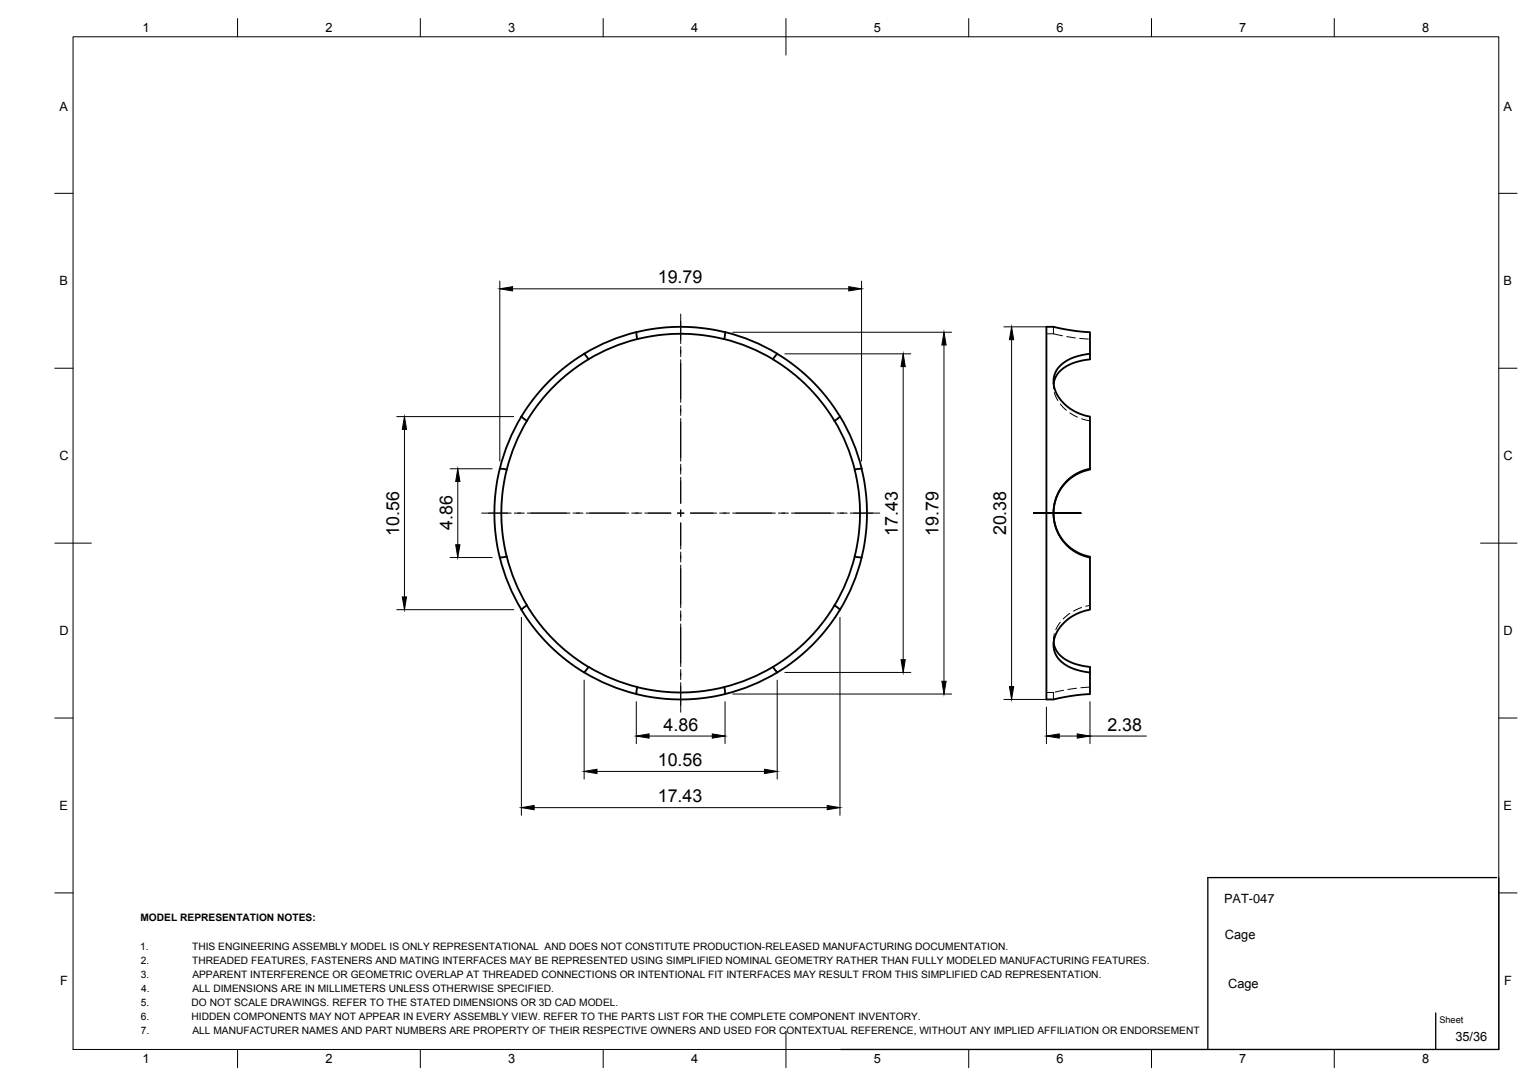
ISO-10303-21;
HEADER;
/* Generated by software containing ST-Developer
 * from STEP Tools, Inc. (www.steptools.com) 
 */

FILE_DESCRIPTION(
/* description */ ('Gravity roller conveyor section'),
/* implementation_level */ '2;1');

FILE_NAME(
/* name */ 'Cage.step',
/* time_stamp */ '2026-11-02T07:43:02-08:00',
/* author */ (''),
/* organization */ (''),
/* preprocessor_version */ 'ST-DEVELOPER v20.2',
/* originating_system */ 'Autodesk Translation Framework v15.17.0.0',
/* authorisation */ '');

FILE_SCHEMA (('AUTOMOTIVE_DESIGN { 1 0 10303 214 3 1 1 }'));
ENDSEC;

DATA;
#10=MECHANICAL_DESIGN_GEOMETRIC_PRESENTATION_REPRESENTATION('',(#562),#13821);
#397=SPHERICAL_SURFACE('',#8542,0.247676);
#398=SPHERICAL_SURFACE('',#8558,0.247676);
#399=SPHERICAL_SURFACE('',#8563,0.247676);
#400=SPHERICAL_SURFACE('',#8568,0.247676);
#401=SPHERICAL_SURFACE('',#8573,0.247676);
#402=SPHERICAL_SURFACE('',#8578,0.247676);
#403=SPHERICAL_SURFACE('',#8583,0.247676);
#404=SPHERICAL_SURFACE('',#8591,0.247676);
#443=B_SPLINE_CURVE_WITH_KNOTS('',3,(#12876,#12877,#12878,#12879,#12880,
#12881,#12882,#12883,#12884,#12885,#12886,#12887,#12888,#12889,#12890,#12891,
#12892,#12893,#12894,#12895,#12896,#12897),.UNSPECIFIED.,.F.,.F.,(4,2,2,
2,2,2,2,2,2,2,4),(0.0473477652366656,0.126350602536658,0.189525903804987,
0.252701205073317,0.313298422430275,0.373895639787233,0.434492857144191,
0.495090074501149,0.558265375769478,0.621440677037807,0.7004435143378),
 .UNSPECIFIED.);
#444=B_SPLINE_CURVE_WITH_KNOTS('',3,(#12901,#12902,#12903,#12904,#12905,
#12906,#12907,#12908,#12909,#12910,#12911,#12912,#12913,#12914,#12915,#12916,
#12917,#12918,#12919,#12920,#12921,#12922),.UNSPECIFIED.,.F.,.F.,(4,2,2,
2,2,2,2,2,2,2,4),(0.0464897534940957,0.0852567806515119,0.170513561303024,
0.246687263103517,0.308657850341199,0.370628437578881,0.432599024816563,
0.494569612054245,0.570743313854739,0.656000094506251,0.694767121663666),
 .UNSPECIFIED.);
#445=B_SPLINE_CURVE_WITH_KNOTS('',3,(#12928,#12929,#12930,#12931,#12932,
#12933,#12934,#12935,#12936,#12937,#12938,#12939,#12940,#12941,#12942,#12943,
#12944,#12945,#12946,#12947,#12948,#12949),.UNSPECIFIED.,.F.,.F.,(4,2,2,
2,2,2,2,2,2,2,4),(0.0464897534940957,0.0852567806515118,0.170513561303024,
0.246687263103517,0.308657850341199,0.370628437578881,0.432599024816563,
0.494569612054245,0.570743313854738,0.65600009450625,0.694767121663666),
 .UNSPECIFIED.);
#446=B_SPLINE_CURVE_WITH_KNOTS('',3,(#12953,#12954,#12955,#12956,#12957,
#12958,#12959,#12960,#12961,#12962,#12963,#12964,#12965,#12966,#12967,#12968,
#12969,#12970,#12971,#12972,#12973,#12974),.UNSPECIFIED.,.F.,.F.,(4,2,2,
2,2,2,2,2,2,2,4),(0.0464897534940957,0.0852567806515119,0.170513561303024,
0.246687263103517,0.308657850341199,0.370628437578881,0.432599024816563,
0.494569612054245,0.570743313854739,0.656000094506251,0.694767121663666),
 .UNSPECIFIED.);
#447=B_SPLINE_CURVE_WITH_KNOTS('',3,(#12978,#12979,#12980,#12981,#12982,
#12983,#12984,#12985,#12986,#12987,#12988,#12989),.UNSPECIFIED.,.F.,.F.,
(4,2,2,2,2,4),(0.0464897534940957,0.0852567806515119,0.170513561303024,
0.246687263103517,0.308657850341199,0.370628437578881),.UNSPECIFIED.);
#448=B_SPLINE_CURVE_WITH_KNOTS('',3,(#12994,#12995,#12996,#12997,#12998,
#12999,#13000,#13001,#13002,#13003,#13004,#13005),.UNSPECIFIED.,.F.,.F.,
(4,2,2,2,2,4),(0.370628437578881,0.432599024816563,0.494569612054245,0.570743313854738,
0.65600009450625,0.694767121663666),.UNSPECIFIED.);
#449=B_SPLINE_CURVE_WITH_KNOTS('',3,(#13009,#13010,#13011,#13012,#13013,
#13014,#13015,#13016,#13017,#13018,#13019,#13020,#13021,#13022,#13023,#13024,
#13025,#13026,#13027,#13028,#13029,#13030),.UNSPECIFIED.,.F.,.F.,(4,2,2,
2,2,2,2,2,2,2,4),(0.0464897534940957,0.0852567806515121,0.170513561303024,
0.246687263103518,0.308657850341199,0.370628437578881,0.432599024816563,
0.494569612054245,0.570743313854738,0.65600009450625,0.694767121663666),
 .UNSPECIFIED.);
#450=B_SPLINE_CURVE_WITH_KNOTS('',3,(#13034,#13035,#13036,#13037,#13038,
#13039,#13040,#13041,#13042,#13043,#13044,#13045,#13046,#13047,#13048,#13049,
#13050,#13051,#13052,#13053,#13054,#13055),.UNSPECIFIED.,.F.,.F.,(4,2,2,
2,2,2,2,2,2,2,4),(0.0464897534940957,0.0852567806515119,0.170513561303024,
0.246687263103517,0.308657850341199,0.370628437578881,0.432599024816563,
0.494569612054245,0.570743313854738,0.65600009450625,0.694767121663667),
 .UNSPECIFIED.);
#451=B_SPLINE_CURVE_WITH_KNOTS('',3,(#13059,#13060,#13061,#13062,#13063,
#13064,#13065,#13066,#13067,#13068,#13069,#13070,#13071,#13072,#13073,#13074,
#13075,#13076,#13077,#13078,#13079,#13080),.UNSPECIFIED.,.F.,.F.,(4,2,2,
2,2,2,2,2,2,2,4),(0.0464897534940957,0.0852567806515119,0.170513561303024,
0.246687263103517,0.308657850341199,0.370628437578881,0.432599024816563,
0.494569612054245,0.570743313854738,0.65600009450625,0.694767121663666),
 .UNSPECIFIED.);
#452=B_SPLINE_CURVE_WITH_KNOTS('',3,(#13084,#13085,#13086,#13087,#13088,
#13089,#13090,#13091,#13092,#13093,#13094,#13095,#13096,#13097,#13098,#13099,
#13100,#13101,#13102,#13103,#13104,#13105),.UNSPECIFIED.,.F.,.F.,(4,2,2,
2,2,2,2,2,2,2,4),(0.0464897534940957,0.0852567806515119,0.170513561303024,
0.246687263103517,0.308657850341199,0.370628437578881,0.432599024816563,
0.494569612054245,0.570743313854739,0.656000094506251,0.694767121663667),
 .UNSPECIFIED.);
#453=B_SPLINE_CURVE_WITH_KNOTS('',3,(#13113,#13114,#13115,#13116,#13117,
#13118,#13119,#13120,#13121,#13122,#13123,#13124,#13125,#13126,#13127,#13128,
#13129,#13130,#13131,#13132,#13133,#13134),.UNSPECIFIED.,.F.,.F.,(4,2,2,
2,2,2,2,2,2,2,4),(0.0473477652366656,0.126350602536658,0.189525903804987,
0.252701205073316,0.313298422430274,0.373895639787232,0.434492857144191,
0.495090074501149,0.558265375769478,0.621440677037807,0.7004435143378),
 .UNSPECIFIED.);
#454=B_SPLINE_CURVE_WITH_KNOTS('',3,(#13142,#13143,#13144,#13145,#13146,
#13147,#13148,#13149,#13150,#13151,#13152,#13153,#13154,#13155,#13156,#13157,
#13158,#13159,#13160,#13161,#13162,#13163),.UNSPECIFIED.,.F.,.F.,(4,2,2,
2,2,2,2,2,2,2,4),(0.0473477652366656,0.126350602536658,0.189525903804987,
0.252701205073317,0.313298422430275,0.373895639787233,0.434492857144191,
0.495090074501149,0.558265375769478,0.621440677037807,0.7004435143378),
 .UNSPECIFIED.);
#455=B_SPLINE_CURVE_WITH_KNOTS('',3,(#13172,#13173,#13174,#13175,#13176,
#13177,#13178,#13179,#13180,#13181,#13182,#13183),.UNSPECIFIED.,.F.,.F.,
(4,2,2,2,2,4),(0.0473477652366656,0.126350602536658,0.189525903804987,0.252701205073316,
0.313298422430275,0.373895639787233),.UNSPECIFIED.);
#456=B_SPLINE_CURVE_WITH_KNOTS('',3,(#13185,#13186,#13187,#13188,#13189,
#13190,#13191,#13192,#13193,#13194,#13195,#13196),.UNSPECIFIED.,.F.,.F.,
(4,2,2,2,2,4),(0.373895639787233,0.434492857144191,0.495090074501149,0.558265375769478,
0.621440677037807,0.7004435143378),.UNSPECIFIED.);
#457=B_SPLINE_CURVE_WITH_KNOTS('',3,(#13203,#13204,#13205,#13206,#13207,
#13208,#13209,#13210,#13211,#13212,#13213,#13214,#13215,#13216,#13217,#13218,
#13219,#13220,#13221,#13222,#13223,#13224),.UNSPECIFIED.,.F.,.F.,(4,2,2,
2,2,2,2,2,2,2,4),(0.0473477652366656,0.126350602536658,0.189525903804987,
0.252701205073316,0.313298422430275,0.373895639787233,0.434492857144191,
0.495090074501149,0.558265375769478,0.621440677037807,0.7004435143378),
 .UNSPECIFIED.);
#458=B_SPLINE_CURVE_WITH_KNOTS('',3,(#13232,#13233,#13234,#13235,#13236,
#13237,#13238,#13239,#13240,#13241,#13242,#13243,#13244,#13245,#13246,#13247,
#13248,#13249,#13250,#13251,#13252,#13253),.UNSPECIFIED.,.F.,.F.,(4,2,2,
2,2,2,2,2,2,2,4),(0.0473477652366656,0.126350602536658,0.189525903804987,
0.252701205073317,0.313298422430275,0.373895639787233,0.434492857144191,
0.495090074501149,0.558265375769478,0.621440677037807,0.7004435143378),
 .UNSPECIFIED.);
#459=B_SPLINE_CURVE_WITH_KNOTS('',3,(#13261,#13262,#13263,#13264,#13265,
#13266,#13267,#13268,#13269,#13270,#13271,#13272,#13273,#13274,#13275,#13276,
#13277,#13278,#13279,#13280,#13281,#13282),.UNSPECIFIED.,.F.,.F.,(4,2,2,
2,2,2,2,2,2,2,4),(0.0473477652366656,0.126350602536658,0.189525903804987,
0.252701205073316,0.313298422430275,0.373895639787233,0.434492857144191,
0.495090074501149,0.558265375769478,0.621440677037807,0.7004435143378),
 .UNSPECIFIED.);
#460=B_SPLINE_CURVE_WITH_KNOTS('',3,(#13291,#13292,#13293,#13294,#13295,
#13296,#13297,#13298,#13299,#13300,#13301,#13302,#13303,#13304,#13305,#13306,
#13307,#13308,#13309,#13310,#13311,#13312),.UNSPECIFIED.,.F.,.F.,(4,2,2,
2,2,2,2,2,2,2,4),(0.0473477652366656,0.126350602536658,0.189525903804987,
0.252701205073317,0.313298422430275,0.373895639787233,0.434492857144191,
0.495090074501149,0.558265375769478,0.621440677037807,0.7004435143378),
 .UNSPECIFIED.);
#487=SHAPE_REPRESENTATION_RELATIONSHIP('SRR','None',#14026,#521);
#521=ADVANCED_BREP_SHAPE_REPRESENTATION('',(#602),#13813);
#562=STYLED_ITEM('',(#14190),#602);
#602=MANIFOLD_SOLID_BREP('Continuous crown cage',#7662);
#682=FACE_BOUND('',#1842,.T.);
#947=PLANE('',#8555);
#948=PLANE('',#8560);
#949=PLANE('',#8565);
#950=PLANE('',#8570);
#951=PLANE('',#8575);
#952=PLANE('',#8580);
#953=PLANE('',#8589);
#954=PLANE('',#8593);
#955=PLANE('',#8594);
#1332=FACE_OUTER_BOUND('',#1824,.T.);
#1333=FACE_OUTER_BOUND('',#1825,.T.);
#1334=FACE_OUTER_BOUND('',#1826,.T.);
#1335=FACE_OUTER_BOUND('',#1827,.T.);
#1336=FACE_OUTER_BOUND('',#1828,.T.);
#1337=FACE_OUTER_BOUND('',#1829,.T.);
#1338=FACE_OUTER_BOUND('',#1830,.T.);
#1339=FACE_OUTER_BOUND('',#1831,.T.);
#1340=FACE_OUTER_BOUND('',#1832,.T.);
#1341=FACE_OUTER_BOUND('',#1833,.T.);
#1342=FACE_OUTER_BOUND('',#1834,.T.);
#1343=FACE_OUTER_BOUND('',#1835,.T.);
#1344=FACE_OUTER_BOUND('',#1836,.T.);
#1345=FACE_OUTER_BOUND('',#1837,.T.);
#1346=FACE_OUTER_BOUND('',#1838,.T.);
#1347=FACE_OUTER_BOUND('',#1839,.T.);
#1348=FACE_OUTER_BOUND('',#1840,.T.);
#1349=FACE_OUTER_BOUND('',#1841,.T.);
#1350=FACE_OUTER_BOUND('',#1843,.T.);
#1824=EDGE_LOOP('',(#6722,#6723,#6724,#6725));
#1825=EDGE_LOOP('',(#6726,#6727,#6728,#6729,#6730,#6731,#6732,#6733,#6734,
#6735,#6736,#6737,#6738,#6739,#6740,#6741,#6742,#6743,#6744,#6745));
#1826=EDGE_LOOP('',(#6746,#6747,#6748,#6749));
#1827=EDGE_LOOP('',(#6750,#6751,#6752,#6753));
#1828=EDGE_LOOP('',(#6754,#6755,#6756,#6757));
#1829=EDGE_LOOP('',(#6758,#6759,#6760,#6761));
#1830=EDGE_LOOP('',(#6762,#6763,#6764,#6765));
#1831=EDGE_LOOP('',(#6766,#6767,#6768,#6769,#6770,#6771));
#1832=EDGE_LOOP('',(#6772,#6773,#6774,#6775));
#1833=EDGE_LOOP('',(#6776,#6777,#6778,#6779));
#1834=EDGE_LOOP('',(#6780,#6781,#6782,#6783));
#1835=EDGE_LOOP('',(#6784,#6785,#6786,#6787));
#1836=EDGE_LOOP('',(#6788,#6789,#6790,#6791));
#1837=EDGE_LOOP('',(#6792,#6793,#6794,#6795));
#1838=EDGE_LOOP('',(#6796,#6797,#6798,#6799,#6800,#6801,#6802,#6803,#6804,
#6805,#6806,#6807,#6808,#6809,#6810,#6811,#6812,#6813,#6814,#6815));
#1839=EDGE_LOOP('',(#6816,#6817,#6818,#6819));
#1840=EDGE_LOOP('',(#6820,#6821,#6822,#6823));
#1841=EDGE_LOOP('',(#6824));
#1842=EDGE_LOOP('',(#6825));
#1843=EDGE_LOOP('',(#6826,#6827,#6828,#6829));
#2550=LINE('',#12991,#3268);
#2551=LINE('',#13287,#3269);
#3268=VECTOR('',#10431,1.019052);
#3269=VECTOR('',#10508,0.980948);
#3512=CIRCLE('',#8543,0.243053047864041);
#3513=CIRCLE('',#8544,0.243053047864041);
#3514=CIRCLE('',#8546,1.019052);
#3515=CIRCLE('',#8547,1.019052);
#3516=CIRCLE('',#8548,1.019052);
#3517=CIRCLE('',#8549,1.019052);
#3518=CIRCLE('',#8550,1.019052);
#3519=CIRCLE('',#8551,1.019052);
#3520=CIRCLE('',#8552,1.019052);
#3521=CIRCLE('',#8553,1.019052);
#3522=CIRCLE('',#8554,1.019052);
#3523=CIRCLE('',#8556,0.980948);
#3524=CIRCLE('',#8557,0.243053047864041);
#3525=CIRCLE('',#8559,0.243053047864041);
#3526=CIRCLE('',#8561,0.980948);
#3527=CIRCLE('',#8562,0.243053047864041);
#3528=CIRCLE('',#8564,0.243053047864041);
#3529=CIRCLE('',#8566,0.980948);
#3530=CIRCLE('',#8567,0.243053047864041);
#3531=CIRCLE('',#8569,0.243053047864041);
#3532=CIRCLE('',#8571,0.980948);
#3533=CIRCLE('',#8572,0.243053047864041);
#3534=CIRCLE('',#8574,0.243053047864041);
#3535=CIRCLE('',#8576,0.980948);
#3536=CIRCLE('',#8577,0.243053047864041);
#3537=CIRCLE('',#8579,0.243053047864041);
#3538=CIRCLE('',#8581,0.980948);
#3539=CIRCLE('',#8582,0.243053047864041);
#3540=CIRCLE('',#8584,0.243053047864041);
#3541=CIRCLE('',#8586,0.980948);
#3542=CIRCLE('',#8587,0.980948);
#3543=CIRCLE('',#8588,0.980948);
#3544=CIRCLE('',#8590,0.243053047864041);
#3545=CIRCLE('',#8592,0.243053047864041);
#4104=VERTEX_POINT('',#12874);
#4105=VERTEX_POINT('',#12875);
#4106=VERTEX_POINT('',#12898);
#4107=VERTEX_POINT('',#12900);
#4108=VERTEX_POINT('',#12925);
#4109=VERTEX_POINT('',#12927);
#4110=VERTEX_POINT('',#12950);
#4111=VERTEX_POINT('',#12952);
#4112=VERTEX_POINT('',#12975);
#4113=VERTEX_POINT('',#12977);
#4114=VERTEX_POINT('',#12990);
#4115=VERTEX_POINT('',#12993);
#4116=VERTEX_POINT('',#13006);
#4117=VERTEX_POINT('',#13008);
#4118=VERTEX_POINT('',#13031);
#4119=VERTEX_POINT('',#13033);
#4120=VERTEX_POINT('',#13056);
#4121=VERTEX_POINT('',#13058);
#4122=VERTEX_POINT('',#13081);
#4123=VERTEX_POINT('',#13083);
#4124=VERTEX_POINT('',#13108);
#4125=VERTEX_POINT('',#13112);
#4126=VERTEX_POINT('',#13137);
#4127=VERTEX_POINT('',#13141);
#4128=VERTEX_POINT('',#13166);
#4129=VERTEX_POINT('',#13170);
#4130=VERTEX_POINT('',#13171);
#4131=VERTEX_POINT('',#13198);
#4132=VERTEX_POINT('',#13202);
#4133=VERTEX_POINT('',#13227);
#4134=VERTEX_POINT('',#13231);
#4135=VERTEX_POINT('',#13256);
#4136=VERTEX_POINT('',#13260);
#4137=VERTEX_POINT('',#13285);
#4138=VERTEX_POINT('',#13288);
#4139=VERTEX_POINT('',#13290);
#4998=EDGE_CURVE('',#4104,#4105,#443,.T.);
#4999=EDGE_CURVE('',#4106,#4104,#3512,.T.);
#5000=EDGE_CURVE('',#4107,#4106,#444,.T.);
#5001=EDGE_CURVE('',#4105,#4107,#3513,.T.);
#5002=EDGE_CURVE('',#4108,#4106,#3514,.T.);
#5003=EDGE_CURVE('',#4108,#4109,#445,.T.);
#5004=EDGE_CURVE('',#4110,#4109,#3515,.T.);
#5005=EDGE_CURVE('',#4110,#4111,#446,.T.);
#5006=EDGE_CURVE('',#4112,#4111,#3516,.T.);
#5007=EDGE_CURVE('',#4112,#4113,#447,.T.);
#5008=EDGE_CURVE('',#4113,#4114,#2550,.T.);
#5009=EDGE_CURVE('',#4114,#4114,#3517,.T.);
#5010=EDGE_CURVE('',#4113,#4115,#448,.T.);
#5011=EDGE_CURVE('',#4116,#4115,#3518,.T.);
#5012=EDGE_CURVE('',#4116,#4117,#449,.T.);
#5013=EDGE_CURVE('',#4118,#4117,#3519,.T.);
#5014=EDGE_CURVE('',#4118,#4119,#450,.T.);
#5015=EDGE_CURVE('',#4120,#4119,#3520,.T.);
#5016=EDGE_CURVE('',#4120,#4121,#451,.T.);
#5017=EDGE_CURVE('',#4122,#4121,#3521,.T.);
#5018=EDGE_CURVE('',#4122,#4123,#452,.T.);
#5019=EDGE_CURVE('',#4107,#4123,#3522,.T.);
#5020=EDGE_CURVE('',#4104,#4124,#3523,.T.);
#5021=EDGE_CURVE('',#4124,#4108,#3524,.T.);
#5022=EDGE_CURVE('',#4125,#4124,#453,.T.);
#5023=EDGE_CURVE('',#4109,#4125,#3525,.T.);
#5024=EDGE_CURVE('',#4125,#4126,#3526,.T.);
#5025=EDGE_CURVE('',#4126,#4110,#3527,.T.);
#5026=EDGE_CURVE('',#4127,#4126,#454,.T.);
#5027=EDGE_CURVE('',#4111,#4127,#3528,.T.);
#5028=EDGE_CURVE('',#4127,#4128,#3529,.T.);
#5029=EDGE_CURVE('',#4128,#4112,#3530,.T.);
#5030=EDGE_CURVE('',#4129,#4130,#455,.T.);
#5031=EDGE_CURVE('',#4115,#4129,#3531,.T.);
#5032=EDGE_CURVE('',#4130,#4128,#456,.T.);
#5033=EDGE_CURVE('',#4129,#4131,#3532,.T.);
#5034=EDGE_CURVE('',#4131,#4116,#3533,.T.);
#5035=EDGE_CURVE('',#4132,#4131,#457,.T.);
#5036=EDGE_CURVE('',#4117,#4132,#3534,.T.);
#5037=EDGE_CURVE('',#4132,#4133,#3535,.T.);
#5038=EDGE_CURVE('',#4133,#4118,#3536,.T.);
#5039=EDGE_CURVE('',#4134,#4133,#458,.T.);
#5040=EDGE_CURVE('',#4119,#4134,#3537,.T.);
#5041=EDGE_CURVE('',#4134,#4135,#3538,.T.);
#5042=EDGE_CURVE('',#4135,#4120,#3539,.T.);
#5043=EDGE_CURVE('',#4136,#4135,#459,.T.);
#5044=EDGE_CURVE('',#4121,#4136,#3540,.T.);
#5045=EDGE_CURVE('',#4137,#4137,#3541,.T.);
#5046=EDGE_CURVE('',#4137,#4130,#2551,.T.);
#5047=EDGE_CURVE('',#4138,#4105,#3542,.T.);
#5048=EDGE_CURVE('',#4138,#4139,#460,.T.);
#5049=EDGE_CURVE('',#4136,#4139,#3543,.T.);
#5050=EDGE_CURVE('',#4123,#4138,#3544,.T.);
#5051=EDGE_CURVE('',#4139,#4122,#3545,.T.);
#6722=ORIENTED_EDGE('',*,*,#4998,.F.);
#6723=ORIENTED_EDGE('',*,*,#4999,.F.);
#6724=ORIENTED_EDGE('',*,*,#5000,.F.);
#6725=ORIENTED_EDGE('',*,*,#5001,.F.);
#6726=ORIENTED_EDGE('',*,*,#5000,.T.);
#6727=ORIENTED_EDGE('',*,*,#5002,.F.);
#6728=ORIENTED_EDGE('',*,*,#5003,.T.);
#6729=ORIENTED_EDGE('',*,*,#5004,.F.);
#6730=ORIENTED_EDGE('',*,*,#5005,.T.);
#6731=ORIENTED_EDGE('',*,*,#5006,.F.);
#6732=ORIENTED_EDGE('',*,*,#5007,.T.);
#6733=ORIENTED_EDGE('',*,*,#5008,.T.);
#6734=ORIENTED_EDGE('',*,*,#5009,.F.);
#6735=ORIENTED_EDGE('',*,*,#5008,.F.);
#6736=ORIENTED_EDGE('',*,*,#5010,.T.);
#6737=ORIENTED_EDGE('',*,*,#5011,.F.);
#6738=ORIENTED_EDGE('',*,*,#5012,.T.);
#6739=ORIENTED_EDGE('',*,*,#5013,.F.);
#6740=ORIENTED_EDGE('',*,*,#5014,.T.);
#6741=ORIENTED_EDGE('',*,*,#5015,.F.);
#6742=ORIENTED_EDGE('',*,*,#5016,.T.);
#6743=ORIENTED_EDGE('',*,*,#5017,.F.);
#6744=ORIENTED_EDGE('',*,*,#5018,.T.);
#6745=ORIENTED_EDGE('',*,*,#5019,.F.);
#6746=ORIENTED_EDGE('',*,*,#4999,.T.);
#6747=ORIENTED_EDGE('',*,*,#5020,.T.);
#6748=ORIENTED_EDGE('',*,*,#5021,.T.);
#6749=ORIENTED_EDGE('',*,*,#5002,.T.);
#6750=ORIENTED_EDGE('',*,*,#5022,.F.);
#6751=ORIENTED_EDGE('',*,*,#5023,.F.);
#6752=ORIENTED_EDGE('',*,*,#5003,.F.);
#6753=ORIENTED_EDGE('',*,*,#5021,.F.);
#6754=ORIENTED_EDGE('',*,*,#5023,.T.);
#6755=ORIENTED_EDGE('',*,*,#5024,.T.);
#6756=ORIENTED_EDGE('',*,*,#5025,.T.);
#6757=ORIENTED_EDGE('',*,*,#5004,.T.);
#6758=ORIENTED_EDGE('',*,*,#5026,.F.);
#6759=ORIENTED_EDGE('',*,*,#5027,.F.);
#6760=ORIENTED_EDGE('',*,*,#5005,.F.);
#6761=ORIENTED_EDGE('',*,*,#5025,.F.);
#6762=ORIENTED_EDGE('',*,*,#5027,.T.);
#6763=ORIENTED_EDGE('',*,*,#5028,.T.);
#6764=ORIENTED_EDGE('',*,*,#5029,.T.);
#6765=ORIENTED_EDGE('',*,*,#5006,.T.);
#6766=ORIENTED_EDGE('',*,*,#5030,.F.);
#6767=ORIENTED_EDGE('',*,*,#5031,.F.);
#6768=ORIENTED_EDGE('',*,*,#5010,.F.);
#6769=ORIENTED_EDGE('',*,*,#5007,.F.);
#6770=ORIENTED_EDGE('',*,*,#5029,.F.);
#6771=ORIENTED_EDGE('',*,*,#5032,.F.);
#6772=ORIENTED_EDGE('',*,*,#5031,.T.);
#6773=ORIENTED_EDGE('',*,*,#5033,.T.);
#6774=ORIENTED_EDGE('',*,*,#5034,.T.);
#6775=ORIENTED_EDGE('',*,*,#5011,.T.);
#6776=ORIENTED_EDGE('',*,*,#5035,.F.);
#6777=ORIENTED_EDGE('',*,*,#5036,.F.);
#6778=ORIENTED_EDGE('',*,*,#5012,.F.);
#6779=ORIENTED_EDGE('',*,*,#5034,.F.);
#6780=ORIENTED_EDGE('',*,*,#5036,.T.);
#6781=ORIENTED_EDGE('',*,*,#5037,.T.);
#6782=ORIENTED_EDGE('',*,*,#5038,.T.);
#6783=ORIENTED_EDGE('',*,*,#5013,.T.);
#6784=ORIENTED_EDGE('',*,*,#5039,.F.);
#6785=ORIENTED_EDGE('',*,*,#5040,.F.);
#6786=ORIENTED_EDGE('',*,*,#5014,.F.);
#6787=ORIENTED_EDGE('',*,*,#5038,.F.);
#6788=ORIENTED_EDGE('',*,*,#5040,.T.);
#6789=ORIENTED_EDGE('',*,*,#5041,.T.);
#6790=ORIENTED_EDGE('',*,*,#5042,.T.);
#6791=ORIENTED_EDGE('',*,*,#5015,.T.);
#6792=ORIENTED_EDGE('',*,*,#5016,.F.);
#6793=ORIENTED_EDGE('',*,*,#5042,.F.);
#6794=ORIENTED_EDGE('',*,*,#5043,.F.);
#6795=ORIENTED_EDGE('',*,*,#5044,.F.);
#6796=ORIENTED_EDGE('',*,*,#5045,.F.);
#6797=ORIENTED_EDGE('',*,*,#5046,.T.);
#6798=ORIENTED_EDGE('',*,*,#5032,.T.);
#6799=ORIENTED_EDGE('',*,*,#5028,.F.);
#6800=ORIENTED_EDGE('',*,*,#5026,.T.);
#6801=ORIENTED_EDGE('',*,*,#5024,.F.);
#6802=ORIENTED_EDGE('',*,*,#5022,.T.);
#6803=ORIENTED_EDGE('',*,*,#5020,.F.);
#6804=ORIENTED_EDGE('',*,*,#4998,.T.);
#6805=ORIENTED_EDGE('',*,*,#5047,.F.);
#6806=ORIENTED_EDGE('',*,*,#5048,.T.);
#6807=ORIENTED_EDGE('',*,*,#5049,.F.);
#6808=ORIENTED_EDGE('',*,*,#5043,.T.);
#6809=ORIENTED_EDGE('',*,*,#5041,.F.);
#6810=ORIENTED_EDGE('',*,*,#5039,.T.);
#6811=ORIENTED_EDGE('',*,*,#5037,.F.);
#6812=ORIENTED_EDGE('',*,*,#5035,.T.);
#6813=ORIENTED_EDGE('',*,*,#5033,.F.);
#6814=ORIENTED_EDGE('',*,*,#5030,.T.);
#6815=ORIENTED_EDGE('',*,*,#5046,.F.);
#6816=ORIENTED_EDGE('',*,*,#5001,.T.);
#6817=ORIENTED_EDGE('',*,*,#5019,.T.);
#6818=ORIENTED_EDGE('',*,*,#5050,.T.);
#6819=ORIENTED_EDGE('',*,*,#5047,.T.);
#6820=ORIENTED_EDGE('',*,*,#5018,.F.);
#6821=ORIENTED_EDGE('',*,*,#5051,.F.);
#6822=ORIENTED_EDGE('',*,*,#5048,.F.);
#6823=ORIENTED_EDGE('',*,*,#5050,.F.);
#6824=ORIENTED_EDGE('',*,*,#5009,.T.);
#6825=ORIENTED_EDGE('',*,*,#5045,.T.);
#6826=ORIENTED_EDGE('',*,*,#5044,.T.);
#6827=ORIENTED_EDGE('',*,*,#5049,.T.);
#6828=ORIENTED_EDGE('',*,*,#5051,.T.);
#6829=ORIENTED_EDGE('',*,*,#5017,.T.);
#7188=CYLINDRICAL_SURFACE('',#8545,1.019052);
#7189=CYLINDRICAL_SURFACE('',#8585,0.980948);
#7533=ADVANCED_FACE('',(#1332),#397,.F.);
#7534=ADVANCED_FACE('',(#1333),#7188,.T.);
#7535=ADVANCED_FACE('',(#1334),#947,.T.);
#7536=ADVANCED_FACE('',(#1335),#398,.F.);
#7537=ADVANCED_FACE('',(#1336),#948,.T.);
#7538=ADVANCED_FACE('',(#1337),#399,.F.);
#7539=ADVANCED_FACE('',(#1338),#949,.T.);
#7540=ADVANCED_FACE('',(#1339),#400,.F.);
#7541=ADVANCED_FACE('',(#1340),#950,.T.);
#7542=ADVANCED_FACE('',(#1341),#401,.F.);
#7543=ADVANCED_FACE('',(#1342),#951,.T.);
#7544=ADVANCED_FACE('',(#1343),#402,.F.);
#7545=ADVANCED_FACE('',(#1344),#952,.T.);
#7546=ADVANCED_FACE('',(#1345),#403,.F.);
#7547=ADVANCED_FACE('',(#1346),#7189,.F.);
#7548=ADVANCED_FACE('',(#1347),#953,.T.);
#7549=ADVANCED_FACE('',(#1348),#404,.F.);
#7550=ADVANCED_FACE('',(#1349,#682),#954,.T.);
#7551=ADVANCED_FACE('',(#1350),#955,.T.);
#7662=CLOSED_SHELL('',(#7533,#7534,#7535,#7536,#7537,#7538,#7539,#7540,
#7541,#7542,#7543,#7544,#7545,#7546,#7547,#7548,#7549,#7550,#7551));
#8541=AXIS2_PLACEMENT_3D('',#12872,#10415,#10416);
#8542=AXIS2_PLACEMENT_3D('',#12873,#10417,#10418);
#8543=AXIS2_PLACEMENT_3D('',#12899,#10419,#10420);
#8544=AXIS2_PLACEMENT_3D('',#12923,#10421,#10422);
#8545=AXIS2_PLACEMENT_3D('',#12924,#10423,#10424);
#8546=AXIS2_PLACEMENT_3D('',#12926,#10425,#10426);
#8547=AXIS2_PLACEMENT_3D('',#12951,#10427,#10428);
#8548=AXIS2_PLACEMENT_3D('',#12976,#10429,#10430);
#8549=AXIS2_PLACEMENT_3D('',#12992,#10432,#10433);
#8550=AXIS2_PLACEMENT_3D('',#13007,#10434,#10435);
#8551=AXIS2_PLACEMENT_3D('',#13032,#10436,#10437);
#8552=AXIS2_PLACEMENT_3D('',#13057,#10438,#10439);
#8553=AXIS2_PLACEMENT_3D('',#13082,#10440,#10441);
#8554=AXIS2_PLACEMENT_3D('',#13106,#10442,#10443);
#8555=AXIS2_PLACEMENT_3D('',#13107,#10444,#10445);
#8556=AXIS2_PLACEMENT_3D('',#13109,#10446,#10447);
#8557=AXIS2_PLACEMENT_3D('',#13110,#10448,#10449);
#8558=AXIS2_PLACEMENT_3D('',#13111,#10450,#10451);
#8559=AXIS2_PLACEMENT_3D('',#13135,#10452,#10453);
#8560=AXIS2_PLACEMENT_3D('',#13136,#10454,#10455);
#8561=AXIS2_PLACEMENT_3D('',#13138,#10456,#10457);
#8562=AXIS2_PLACEMENT_3D('',#13139,#10458,#10459);
#8563=AXIS2_PLACEMENT_3D('',#13140,#10460,#10461);
#8564=AXIS2_PLACEMENT_3D('',#13164,#10462,#10463);
#8565=AXIS2_PLACEMENT_3D('',#13165,#10464,#10465);
#8566=AXIS2_PLACEMENT_3D('',#13167,#10466,#10467);
#8567=AXIS2_PLACEMENT_3D('',#13168,#10468,#10469);
#8568=AXIS2_PLACEMENT_3D('',#13169,#10470,#10471);
#8569=AXIS2_PLACEMENT_3D('',#13184,#10472,#10473);
#8570=AXIS2_PLACEMENT_3D('',#13197,#10474,#10475);
#8571=AXIS2_PLACEMENT_3D('',#13199,#10476,#10477);
#8572=AXIS2_PLACEMENT_3D('',#13200,#10478,#10479);
#8573=AXIS2_PLACEMENT_3D('',#13201,#10480,#10481);
#8574=AXIS2_PLACEMENT_3D('',#13225,#10482,#10483);
#8575=AXIS2_PLACEMENT_3D('',#13226,#10484,#10485);
#8576=AXIS2_PLACEMENT_3D('',#13228,#10486,#10487);
#8577=AXIS2_PLACEMENT_3D('',#13229,#10488,#10489);
#8578=AXIS2_PLACEMENT_3D('',#13230,#10490,#10491);
#8579=AXIS2_PLACEMENT_3D('',#13254,#10492,#10493);
#8580=AXIS2_PLACEMENT_3D('',#13255,#10494,#10495);
#8581=AXIS2_PLACEMENT_3D('',#13257,#10496,#10497);
#8582=AXIS2_PLACEMENT_3D('',#13258,#10498,#10499);
#8583=AXIS2_PLACEMENT_3D('',#13259,#10500,#10501);
#8584=AXIS2_PLACEMENT_3D('',#13283,#10502,#10503);
#8585=AXIS2_PLACEMENT_3D('',#13284,#10504,#10505);
#8586=AXIS2_PLACEMENT_3D('',#13286,#10506,#10507);
#8587=AXIS2_PLACEMENT_3D('',#13289,#10509,#10510);
#8588=AXIS2_PLACEMENT_3D('',#13313,#10511,#10512);
#8589=AXIS2_PLACEMENT_3D('',#13314,#10513,#10514);
#8590=AXIS2_PLACEMENT_3D('',#13315,#10515,#10516);
#8591=AXIS2_PLACEMENT_3D('',#13316,#10517,#10518);
#8592=AXIS2_PLACEMENT_3D('',#13317,#10519,#10520);
#8593=AXIS2_PLACEMENT_3D('',#13318,#10521,#10522);
#8594=AXIS2_PLACEMENT_3D('',#13319,#10523,#10524);
#10415=DIRECTION('axis',(0.,0.,1.));
#10416=DIRECTION('refdir',(1.,0.,0.));
#10417=DIRECTION('center_axis',(0.,0.,1.));
#10418=DIRECTION('ref_axis',(1.,0.,0.));
#10419=DIRECTION('center_axis',(0.,-1.,0.));
#10420=DIRECTION('ref_axis',(0.,0.,-1.));
#10421=DIRECTION('center_axis',(0.,-1.,0.));
#10422=DIRECTION('ref_axis',(0.,0.,-1.));
#10423=DIRECTION('center_axis',(0.,1.,0.));
#10424=DIRECTION('ref_axis',(1.,0.,0.));
#10425=DIRECTION('center_axis',(0.,1.,0.));
#10426=DIRECTION('ref_axis',(1.,0.,0.));
#10427=DIRECTION('center_axis',(0.,1.,0.));
#10428=DIRECTION('ref_axis',(1.,0.,0.));
#10429=DIRECTION('center_axis',(0.,1.,0.));
#10430=DIRECTION('ref_axis',(1.,0.,0.));
#10431=DIRECTION('',(0.,-1.,0.));
#10432=DIRECTION('center_axis',(0.,-1.,0.));
#10433=DIRECTION('ref_axis',(1.,0.,0.));
#10434=DIRECTION('center_axis',(0.,1.,0.));
#10435=DIRECTION('ref_axis',(1.,0.,0.));
#10436=DIRECTION('center_axis',(0.,1.,0.));
#10437=DIRECTION('ref_axis',(1.,0.,0.));
#10438=DIRECTION('center_axis',(0.,1.,0.));
#10439=DIRECTION('ref_axis',(1.,0.,0.));
#10440=DIRECTION('center_axis',(0.,1.,0.));
#10441=DIRECTION('ref_axis',(1.,0.,0.));
#10442=DIRECTION('center_axis',(0.,1.,0.));
#10443=DIRECTION('ref_axis',(1.,0.,0.));
#10444=DIRECTION('center_axis',(0.,1.,0.));
#10445=DIRECTION('ref_axis',(1.,0.,0.));
#10446=DIRECTION('center_axis',(0.,-1.,0.));
#10447=DIRECTION('ref_axis',(1.,0.,0.));
#10448=DIRECTION('center_axis',(0.,-1.,0.));
#10449=DIRECTION('ref_axis',(0.,0.,-1.));
#10450=DIRECTION('center_axis',(6.12323399573677E-17,0.,1.));
#10451=DIRECTION('ref_axis',(1.,0.,0.));
#10452=DIRECTION('center_axis',(0.,-1.,0.));
#10453=DIRECTION('ref_axis',(0.,0.,-1.));
#10454=DIRECTION('center_axis',(0.,1.,0.));
#10455=DIRECTION('ref_axis',(1.,0.,0.));
#10456=DIRECTION('center_axis',(0.,-1.,0.));
#10457=DIRECTION('ref_axis',(1.,0.,0.));
#10458=DIRECTION('center_axis',(0.,-1.,0.));
#10459=DIRECTION('ref_axis',(0.,0.,-1.));
#10460=DIRECTION('center_axis',(0.,0.,1.));
#10461=DIRECTION('ref_axis',(1.,0.,0.));
#10462=DIRECTION('center_axis',(0.,-1.,0.));
#10463=DIRECTION('ref_axis',(0.,0.,-1.));
#10464=DIRECTION('center_axis',(0.,1.,0.));
#10465=DIRECTION('ref_axis',(1.,0.,0.));
#10466=DIRECTION('center_axis',(0.,-1.,0.));
#10467=DIRECTION('ref_axis',(1.,0.,0.));
#10468=DIRECTION('center_axis',(0.,-1.,0.));
#10469=DIRECTION('ref_axis',(0.,0.,-1.));
#10470=DIRECTION('center_axis',(0.,0.,1.));
#10471=DIRECTION('ref_axis',(1.,0.,0.));
#10472=DIRECTION('center_axis',(0.,-1.,0.));
#10473=DIRECTION('ref_axis',(0.,0.,-1.));
#10474=DIRECTION('center_axis',(0.,1.,0.));
#10475=DIRECTION('ref_axis',(1.,0.,0.));
#10476=DIRECTION('center_axis',(0.,-1.,0.));
#10477=DIRECTION('ref_axis',(1.,0.,0.));
#10478=DIRECTION('center_axis',(0.,-1.,0.));
#10479=DIRECTION('ref_axis',(0.,0.,-1.));
#10480=DIRECTION('center_axis',(0.,0.,1.));
#10481=DIRECTION('ref_axis',(1.,0.,0.));
#10482=DIRECTION('center_axis',(0.,-1.,0.));
#10483=DIRECTION('ref_axis',(0.,0.,-1.));
#10484=DIRECTION('center_axis',(0.,1.,0.));
#10485=DIRECTION('ref_axis',(1.,0.,0.));
#10486=DIRECTION('center_axis',(0.,-1.,0.));
#10487=DIRECTION('ref_axis',(1.,0.,0.));
#10488=DIRECTION('center_axis',(0.,-1.,0.));
#10489=DIRECTION('ref_axis',(0.,0.,-1.));
#10490=DIRECTION('center_axis',(6.12323399573676E-17,0.,1.));
#10491=DIRECTION('ref_axis',(1.,0.,0.));
#10492=DIRECTION('center_axis',(0.,-1.,0.));
#10493=DIRECTION('ref_axis',(0.,0.,-1.));
#10494=DIRECTION('center_axis',(0.,1.,0.));
#10495=DIRECTION('ref_axis',(1.,0.,0.));
#10496=DIRECTION('center_axis',(0.,-1.,0.));
#10497=DIRECTION('ref_axis',(1.,0.,0.));
#10498=DIRECTION('center_axis',(0.,-1.,0.));
#10499=DIRECTION('ref_axis',(0.,0.,-1.));
#10500=DIRECTION('center_axis',(0.,0.,1.));
#10501=DIRECTION('ref_axis',(1.,0.,0.));
#10502=DIRECTION('center_axis',(0.,-1.,0.));
#10503=DIRECTION('ref_axis',(0.,0.,-1.));
#10504=DIRECTION('center_axis',(0.,1.,0.));
#10505=DIRECTION('ref_axis',(1.,0.,0.));
#10506=DIRECTION('center_axis',(0.,1.,0.));
#10507=DIRECTION('ref_axis',(1.,0.,0.));
#10508=DIRECTION('',(0.,1.,0.));
#10509=DIRECTION('center_axis',(0.,-1.,0.));
#10510=DIRECTION('ref_axis',(1.,0.,0.));
#10511=DIRECTION('center_axis',(0.,-1.,0.));
#10512=DIRECTION('ref_axis',(1.,0.,0.));
#10513=DIRECTION('center_axis',(0.,1.,0.));
#10514=DIRECTION('ref_axis',(1.,0.,0.));
#10515=DIRECTION('center_axis',(0.,-1.,0.));
#10516=DIRECTION('ref_axis',(0.,0.,-1.));
#10517=DIRECTION('center_axis',(0.,0.,1.));
#10518=DIRECTION('ref_axis',(1.,0.,0.));
#10519=DIRECTION('center_axis',(0.,-1.,0.));
#10520=DIRECTION('ref_axis',(0.,0.,-1.));
#10521=DIRECTION('center_axis',(0.,-1.,0.));
#10522=DIRECTION('ref_axis',(-1.,0.,0.));
#10523=DIRECTION('center_axis',(0.,1.,0.));
#10524=DIRECTION('ref_axis',(1.,0.,0.));
#12872=CARTESIAN_POINT('',(0.,0.,0.));
#12873=CARTESIAN_POINT('Origin',(0.707106781186547,0.,0.707106781186548));
#12874=CARTESIAN_POINT('',(0.504455939115715,-0.04763,0.841298510752802));
#12875=CARTESIAN_POINT('',(0.841298510752802,-0.04763,0.504455939115715));
#12876=CARTESIAN_POINT('Ctrl Pts',(0.504455939115715,-0.04763,0.841298510752802));
#12877=CARTESIAN_POINT('Ctrl Pts',(0.508899795931835,-0.0740444353928835,
0.838633903678357));
#12878=CARTESIAN_POINT('Ctrl Pts',(0.517157748491652,-0.0999305678883309,
0.833661031856294));
#12879=CARTESIAN_POINT('Ctrl Pts',(0.537715343527944,-0.142345102874864,
0.820511285096538));
#12880=CARTESIAN_POINT('Ctrl Pts',(0.548874290046456,-0.159766064500479,
0.813159949759));
#12881=CARTESIAN_POINT('Ctrl Pts',(0.573915184558107,-0.190326085855194,
0.795684265985089));
#12882=CARTESIAN_POINT('Ctrl Pts',(0.587792702767295,-0.203463743702801,
0.78555112003688));
#12883=CARTESIAN_POINT('Ctrl Pts',(0.615966552324775,-0.224161999508995,
0.763642258217233));
#12884=CARTESIAN_POINT('Ctrl Pts',(0.631684198665438,-0.232861760990032,
0.750785745543687));
#12885=CARTESIAN_POINT('Ctrl Pts',(0.663382628119203,-0.244251601209411,
0.722929908501543));
#12886=CARTESIAN_POINT('Ctrl Pts',(0.679352081686668,-0.246942143572133,
0.707917883896095));
#12887=CARTESIAN_POINT('Ctrl Pts',(0.707917883896095,-0.246942143572133,
0.679352081686668));
#12888=CARTESIAN_POINT('Ctrl Pts',(0.722929908501543,-0.244251601209411,
0.663382628119203));
#12889=CARTESIAN_POINT('Ctrl Pts',(0.750785745543687,-0.232861760990032,
0.631684198665439));
#12890=CARTESIAN_POINT('Ctrl Pts',(0.763642258217232,-0.224161999508995,
0.615966552324775));
#12891=CARTESIAN_POINT('Ctrl Pts',(0.78555112003688,-0.203463743702801,
0.587792702767295));
#12892=CARTESIAN_POINT('Ctrl Pts',(0.795684265985088,-0.190326085855194,
0.573915184558108));
#12893=CARTESIAN_POINT('Ctrl Pts',(0.813159949759,-0.15976606450048,0.548874290046456));
#12894=CARTESIAN_POINT('Ctrl Pts',(0.820511285096538,-0.142345102874864,
0.537715343527944));
#12895=CARTESIAN_POINT('Ctrl Pts',(0.833661031856294,-0.099930567888331,
0.517157748491653));
#12896=CARTESIAN_POINT('Ctrl Pts',(0.838633903678357,-0.0740444353928835,
0.508899795931835));
#12897=CARTESIAN_POINT('Ctrl Pts',(0.841298510752801,-0.0476299999999999,
0.504455939115715));
#12898=CARTESIAN_POINT('',(0.528110872004958,-0.04763,0.871530771444223));
#12899=CARTESIAN_POINT('Origin',(0.707106781186547,-0.04763,0.707106781186548));
#12900=CARTESIAN_POINT('',(0.871530771444223,-0.04763,0.528110872004959));
#12901=CARTESIAN_POINT('Ctrl Pts',(0.871530771444223,-0.0476300000000001,
0.528110872004958));
#12902=CARTESIAN_POINT('Ctrl Pts',(0.87014664509073,-0.0609922781173483,
0.530395067942936));
#12903=CARTESIAN_POINT('Ctrl Pts',(0.868149331745851,-0.0742967091364493,
0.533674141594226));
#12904=CARTESIAN_POINT('Ctrl Pts',(0.85981294420286,-0.115492077056649,
0.54708917182331));
#12905=CARTESIAN_POINT('Ctrl Pts',(0.850993704737257,-0.141695629206859,
0.560922177770136));
#12906=CARTESIAN_POINT('Ctrl Pts',(0.830754510485543,-0.181890537957859,
0.590422647829571));
#12907=CARTESIAN_POINT('Ctrl Pts',(0.816896541396381,-0.201072148666545,
0.609616703125488));
#12908=CARTESIAN_POINT('Ctrl Pts',(0.792310597819928,-0.223955109275652,
0.641117951819998));
#12909=CARTESIAN_POINT('Ctrl Pts',(0.779109323683612,-0.232742381310829,
0.657208095763053));
#12910=CARTESIAN_POINT('Ctrl Pts',(0.750552691816206,-0.244234834628584,
0.68964083160521));
#12911=CARTESIAN_POINT('Ctrl Pts',(0.735185187071673,-0.246942143572133,
0.705971972091755));
#12912=CARTESIAN_POINT('Ctrl Pts',(0.705971972091754,-0.246942143572133,
0.735185187071673));
#12913=CARTESIAN_POINT('Ctrl Pts',(0.689640831605209,-0.244234834628584,
0.750552691816206));
#12914=CARTESIAN_POINT('Ctrl Pts',(0.657208095763052,-0.232742381310829,
0.779109323683612));
#12915=CARTESIAN_POINT('Ctrl Pts',(0.641117951819998,-0.223955109275652,
0.792310597819928));
#12916=CARTESIAN_POINT('Ctrl Pts',(0.609616703125487,-0.201072148666545,
0.816896541396382));
#12917=CARTESIAN_POINT('Ctrl Pts',(0.590422647829571,-0.181890537957858,
0.830754510485544));
#12918=CARTESIAN_POINT('Ctrl Pts',(0.560922177770135,-0.141695629206858,
0.850993704737257));
#12919=CARTESIAN_POINT('Ctrl Pts',(0.547089171823309,-0.115492077056649,
0.859812944202861));
#12920=CARTESIAN_POINT('Ctrl Pts',(0.533674141594226,-0.0742967091364491,
0.868149331745852));
#12921=CARTESIAN_POINT('Ctrl Pts',(0.530395067942936,-0.0609922781173483,
0.870146645090731));
#12922=CARTESIAN_POINT('Ctrl Pts',(0.528110872004958,-0.0476300000000001,
0.871530771444223));
#12923=CARTESIAN_POINT('Origin',(0.707106781186547,-0.04763,0.707106781186548));
#12924=CARTESIAN_POINT('Origin',(0.,-0.166705,0.));
#12925=CARTESIAN_POINT('',(0.242834539687906,-0.04763,0.989696097314));
#12926=CARTESIAN_POINT('Origin',(0.,-0.04763,0.));
#12927=CARTESIAN_POINT('',(-0.242834539687907,-0.04763,0.989696097314));
#12928=CARTESIAN_POINT('Ctrl Pts',(0.242834539687906,-0.04763,0.989696097314));
#12929=CARTESIAN_POINT('Ctrl Pts',(0.24024064412003,-0.0609922781173483,
0.990332542620729));
#12930=CARTESIAN_POINT('Ctrl Pts',(0.236509675094874,-0.0742967091364492,
0.991238884025248));
#12931=CARTESIAN_POINT('Ctrl Pts',(0.221129100087819,-0.115492077056649,
0.994830026707808));
#12932=CARTESIAN_POINT('Ctrl Pts',(0.205111543747588,-0.141695629206859,
0.998375294985966));
#12933=CARTESIAN_POINT('Ctrl Pts',(0.169940289819232,-0.181890537957859,
1.00492400591205));
#12934=CARTESIAN_POINT('Ctrl Pts',(0.1465689792446,-0.201072148666545,1.00869718865384));
#12935=CARTESIAN_POINT('Ctrl Pts',(0.106909345252087,-0.223955109275652,
1.01358704779679));
#12936=CARTESIAN_POINT('Ctrl Pts',(0.0861971848975941,-0.232742381310829,
1.0156297872271));
#12937=CARTESIAN_POINT('Ctrl Pts',(0.0430711894098822,-0.244234834628584,
1.01837060663223));
#12938=CARTESIAN_POINT('Ctrl Pts',(0.0206568624125605,-0.246942143572133,
1.019052));
#12939=CARTESIAN_POINT('Ctrl Pts',(-0.0206568624125608,-0.246942143572133,
1.019052));
#12940=CARTESIAN_POINT('Ctrl Pts',(-0.0430711894098825,-0.244234834628584,
1.01837060663223));
#12941=CARTESIAN_POINT('Ctrl Pts',(-0.0861971848975943,-0.232742381310829,
1.0156297872271));
#12942=CARTESIAN_POINT('Ctrl Pts',(-0.106909345252088,-0.223955109275652,
1.01358704779679));
#12943=CARTESIAN_POINT('Ctrl Pts',(-0.1465689792446,-0.201072148666545,
1.00869718865384));
#12944=CARTESIAN_POINT('Ctrl Pts',(-0.169940289819232,-0.181890537957859,
1.00492400591205));
#12945=CARTESIAN_POINT('Ctrl Pts',(-0.205111543747588,-0.141695629206859,
0.998375294985966));
#12946=CARTESIAN_POINT('Ctrl Pts',(-0.221129100087819,-0.115492077056649,
0.994830026707808));
#12947=CARTESIAN_POINT('Ctrl Pts',(-0.236509675094875,-0.0742967091364493,
0.991238884025248));
#12948=CARTESIAN_POINT('Ctrl Pts',(-0.24024064412003,-0.0609922781173483,
0.990332542620729));
#12949=CARTESIAN_POINT('Ctrl Pts',(-0.242834539687907,-0.04763,0.989696097314));
#12950=CARTESIAN_POINT('',(-0.528110872004959,-0.04763,0.871530771444223));
#12951=CARTESIAN_POINT('Origin',(0.,-0.04763,0.));
#12952=CARTESIAN_POINT('',(-0.871530771444223,-0.04763,0.528110872004958));
#12953=CARTESIAN_POINT('Ctrl Pts',(-0.528110872004958,-0.0476300000000001,
0.871530771444223));
#12954=CARTESIAN_POINT('Ctrl Pts',(-0.530395067942936,-0.0609922781173484,
0.87014664509073));
#12955=CARTESIAN_POINT('Ctrl Pts',(-0.533674141594226,-0.0742967091364493,
0.868149331745851));
#12956=CARTESIAN_POINT('Ctrl Pts',(-0.54708917182331,-0.115492077056649,
0.85981294420286));
#12957=CARTESIAN_POINT('Ctrl Pts',(-0.560922177770136,-0.141695629206859,
0.850993704737257));
#12958=CARTESIAN_POINT('Ctrl Pts',(-0.590422647829571,-0.181890537957859,
0.830754510485543));
#12959=CARTESIAN_POINT('Ctrl Pts',(-0.609616703125488,-0.201072148666545,
0.816896541396381));
#12960=CARTESIAN_POINT('Ctrl Pts',(-0.641117951819998,-0.223955109275652,
0.792310597819928));
#12961=CARTESIAN_POINT('Ctrl Pts',(-0.657208095763053,-0.232742381310829,
0.779109323683611));
#12962=CARTESIAN_POINT('Ctrl Pts',(-0.68964083160521,-0.244234834628584,
0.750552691816205));
#12963=CARTESIAN_POINT('Ctrl Pts',(-0.705971972091755,-0.246942143572133,
0.735185187071673));
#12964=CARTESIAN_POINT('Ctrl Pts',(-0.735185187071673,-0.246942143572133,
0.705971972091754));
#12965=CARTESIAN_POINT('Ctrl Pts',(-0.750552691816206,-0.244234834628584,
0.689640831605209));
#12966=CARTESIAN_POINT('Ctrl Pts',(-0.779109323683612,-0.232742381310829,
0.657208095763052));
#12967=CARTESIAN_POINT('Ctrl Pts',(-0.792310597819928,-0.223955109275652,
0.641117951819998));
#12968=CARTESIAN_POINT('Ctrl Pts',(-0.816896541396382,-0.201072148666545,
0.609616703125487));
#12969=CARTESIAN_POINT('Ctrl Pts',(-0.830754510485544,-0.181890537957858,
0.590422647829571));
#12970=CARTESIAN_POINT('Ctrl Pts',(-0.850993704737257,-0.141695629206858,
0.560922177770135));
#12971=CARTESIAN_POINT('Ctrl Pts',(-0.859812944202861,-0.115492077056649,
0.547089171823309));
#12972=CARTESIAN_POINT('Ctrl Pts',(-0.868149331745852,-0.0742967091364491,
0.533674141594226));
#12973=CARTESIAN_POINT('Ctrl Pts',(-0.870146645090731,-0.0609922781173483,
0.530395067942936));
#12974=CARTESIAN_POINT('Ctrl Pts',(-0.871530771444223,-0.04763,0.528110872004958));
#12975=CARTESIAN_POINT('',(-0.989696097314,-0.04763,0.242834539687906));
#12976=CARTESIAN_POINT('Origin',(0.,-0.04763,0.));
#12977=CARTESIAN_POINT('',(-1.019052,-0.246942143572133,1.248489836334E-16));
#12978=CARTESIAN_POINT('Ctrl Pts',(-0.989696097314,-0.04763,0.242834539687906));
#12979=CARTESIAN_POINT('Ctrl Pts',(-0.990332542620729,-0.0609922781173483,
0.24024064412003));
#12980=CARTESIAN_POINT('Ctrl Pts',(-0.991238884025248,-0.0742967091364492,
0.236509675094874));
#12981=CARTESIAN_POINT('Ctrl Pts',(-0.994830026707808,-0.115492077056649,
0.221129100087819));
#12982=CARTESIAN_POINT('Ctrl Pts',(-0.998375294985966,-0.141695629206859,
0.205111543747588));
#12983=CARTESIAN_POINT('Ctrl Pts',(-1.00492400591205,-0.181890537957859,
0.169940289819232));
#12984=CARTESIAN_POINT('Ctrl Pts',(-1.00869718865384,-0.201072148666545,
0.1465689792446));
#12985=CARTESIAN_POINT('Ctrl Pts',(-1.01358704779679,-0.223955109275652,
0.106909345252088));
#12986=CARTESIAN_POINT('Ctrl Pts',(-1.0156297872271,-0.232742381310829,
0.0861971848975944));
#12987=CARTESIAN_POINT('Ctrl Pts',(-1.01837060663223,-0.244234834628584,
0.0430711894098825));
#12988=CARTESIAN_POINT('Ctrl Pts',(-1.019052,-0.246942143572133,0.0206568624125608));
#12989=CARTESIAN_POINT('Ctrl Pts',(-1.019052,-0.246942143572133,1.2490009027033E-16));
#12990=CARTESIAN_POINT('',(-1.019052,-0.28578,1.24797876996471E-16));
#12991=CARTESIAN_POINT('',(-1.019052,-0.166705,1.24797876996471E-16));
#12992=CARTESIAN_POINT('Origin',(0.,-0.28578,0.));
#12993=CARTESIAN_POINT('',(-0.989696097314,-0.04763,-0.242834539687906));
#12994=CARTESIAN_POINT('Ctrl Pts',(-1.019052,-0.246942143572133,1.2490009027033E-16));
#12995=CARTESIAN_POINT('Ctrl Pts',(-1.019052,-0.246942143572133,-0.0206568624125605));
#12996=CARTESIAN_POINT('Ctrl Pts',(-1.01837060663223,-0.244234834628584,
-0.0430711894098822));
#12997=CARTESIAN_POINT('Ctrl Pts',(-1.0156297872271,-0.232742381310829,
-0.0861971848975941));
#12998=CARTESIAN_POINT('Ctrl Pts',(-1.01358704779679,-0.223955109275652,
-0.106909345252087));
#12999=CARTESIAN_POINT('Ctrl Pts',(-1.00869718865384,-0.201072148666546,
-0.1465689792446));
#13000=CARTESIAN_POINT('Ctrl Pts',(-1.00492400591205,-0.181890537957859,
-0.169940289819232));
#13001=CARTESIAN_POINT('Ctrl Pts',(-0.998375294985966,-0.141695629206859,
-0.205111543747588));
#13002=CARTESIAN_POINT('Ctrl Pts',(-0.994830026707808,-0.11549207705665,
-0.221129100087819));
#13003=CARTESIAN_POINT('Ctrl Pts',(-0.991238884025248,-0.0742967091364495,
-0.236509675094874));
#13004=CARTESIAN_POINT('Ctrl Pts',(-0.990332542620729,-0.0609922781173484,
-0.24024064412003));
#13005=CARTESIAN_POINT('Ctrl Pts',(-0.989696097314,-0.0476300000000001,
-0.242834539687907));
#13006=CARTESIAN_POINT('',(-0.871530771444223,-0.04763,-0.528110872004958));
#13007=CARTESIAN_POINT('Origin',(0.,-0.04763,0.));
#13008=CARTESIAN_POINT('',(-0.528110872004958,-0.04763,-0.871530771444223));
#13009=CARTESIAN_POINT('Ctrl Pts',(-0.871530771444223,-0.0476300000000001,
-0.528110872004958));
#13010=CARTESIAN_POINT('Ctrl Pts',(-0.87014664509073,-0.0609922781173484,
-0.530395067942936));
#13011=CARTESIAN_POINT('Ctrl Pts',(-0.868149331745851,-0.0742967091364494,
-0.533674141594226));
#13012=CARTESIAN_POINT('Ctrl Pts',(-0.85981294420286,-0.115492077056649,
-0.54708917182331));
#13013=CARTESIAN_POINT('Ctrl Pts',(-0.850993704737257,-0.141695629206859,
-0.560922177770136));
#13014=CARTESIAN_POINT('Ctrl Pts',(-0.830754510485543,-0.181890537957859,
-0.590422647829571));
#13015=CARTESIAN_POINT('Ctrl Pts',(-0.816896541396381,-0.201072148666546,
-0.609616703125488));
#13016=CARTESIAN_POINT('Ctrl Pts',(-0.792310597819928,-0.223955109275652,
-0.641117951819999));
#13017=CARTESIAN_POINT('Ctrl Pts',(-0.779109323683611,-0.232742381310829,
-0.657208095763053));
#13018=CARTESIAN_POINT('Ctrl Pts',(-0.750552691816205,-0.244234834628584,
-0.68964083160521));
#13019=CARTESIAN_POINT('Ctrl Pts',(-0.735185187071673,-0.246942143572133,
-0.705971972091755));
#13020=CARTESIAN_POINT('Ctrl Pts',(-0.705971972091754,-0.246942143572133,
-0.735185187071673));
#13021=CARTESIAN_POINT('Ctrl Pts',(-0.68964083160521,-0.244234834628584,
-0.750552691816206));
#13022=CARTESIAN_POINT('Ctrl Pts',(-0.657208095763052,-0.232742381310829,
-0.779109323683612));
#13023=CARTESIAN_POINT('Ctrl Pts',(-0.641117951819998,-0.223955109275652,
-0.792310597819928));
#13024=CARTESIAN_POINT('Ctrl Pts',(-0.609616703125488,-0.201072148666545,
-0.816896541396381));
#13025=CARTESIAN_POINT('Ctrl Pts',(-0.590422647829571,-0.181890537957859,
-0.830754510485543));
#13026=CARTESIAN_POINT('Ctrl Pts',(-0.560922177770136,-0.141695629206859,
-0.850993704737257));
#13027=CARTESIAN_POINT('Ctrl Pts',(-0.54708917182331,-0.115492077056649,
-0.85981294420286));
#13028=CARTESIAN_POINT('Ctrl Pts',(-0.533674141594226,-0.0742967091364494,
-0.868149331745852));
#13029=CARTESIAN_POINT('Ctrl Pts',(-0.530395067942936,-0.0609922781173484,
-0.870146645090731));
#13030=CARTESIAN_POINT('Ctrl Pts',(-0.528110872004958,-0.0476300000000001,
-0.871530771444223));
#13031=CARTESIAN_POINT('',(-0.242834539687906,-0.04763,-0.989696097314));
#13032=CARTESIAN_POINT('Origin',(0.,-0.04763,0.));
#13033=CARTESIAN_POINT('',(0.242834539687906,-0.04763,-0.989696097314));
#13034=CARTESIAN_POINT('Ctrl Pts',(-0.242834539687907,-0.04763,-0.989696097314));
#13035=CARTESIAN_POINT('Ctrl Pts',(-0.24024064412003,-0.0609922781173483,
-0.990332542620729));
#13036=CARTESIAN_POINT('Ctrl Pts',(-0.236509675094874,-0.0742967091364493,
-0.991238884025248));
#13037=CARTESIAN_POINT('Ctrl Pts',(-0.221129100087819,-0.115492077056649,
-0.994830026707808));
#13038=CARTESIAN_POINT('Ctrl Pts',(-0.205111543747588,-0.141695629206859,
-0.998375294985966));
#13039=CARTESIAN_POINT('Ctrl Pts',(-0.169940289819232,-0.181890537957859,
-1.00492400591205));
#13040=CARTESIAN_POINT('Ctrl Pts',(-0.1465689792446,-0.201072148666545,
-1.00869718865384));
#13041=CARTESIAN_POINT('Ctrl Pts',(-0.106909345252087,-0.223955109275652,
-1.01358704779679));
#13042=CARTESIAN_POINT('Ctrl Pts',(-0.0861971848975942,-0.232742381310829,
-1.0156297872271));
#13043=CARTESIAN_POINT('Ctrl Pts',(-0.0430711894098823,-0.244234834628584,
-1.01837060663223));
#13044=CARTESIAN_POINT('Ctrl Pts',(-0.0206568624125606,-0.246942143572133,
-1.019052));
#13045=CARTESIAN_POINT('Ctrl Pts',(0.0206568624125607,-0.246942143572133,
-1.019052));
#13046=CARTESIAN_POINT('Ctrl Pts',(0.0430711894098824,-0.244234834628584,
-1.01837060663223));
#13047=CARTESIAN_POINT('Ctrl Pts',(0.0861971848975943,-0.232742381310829,
-1.0156297872271));
#13048=CARTESIAN_POINT('Ctrl Pts',(0.106909345252088,-0.223955109275652,
-1.01358704779679));
#13049=CARTESIAN_POINT('Ctrl Pts',(0.1465689792446,-0.201072148666545,-1.00869718865384));
#13050=CARTESIAN_POINT('Ctrl Pts',(0.169940289819232,-0.181890537957859,
-1.00492400591205));
#13051=CARTESIAN_POINT('Ctrl Pts',(0.205111543747588,-0.141695629206859,
-0.998375294985966));
#13052=CARTESIAN_POINT('Ctrl Pts',(0.221129100087819,-0.115492077056649,
-0.994830026707808));
#13053=CARTESIAN_POINT('Ctrl Pts',(0.236509675094874,-0.0742967091364493,
-0.991238884025248));
#13054=CARTESIAN_POINT('Ctrl Pts',(0.24024064412003,-0.0609922781173484,
-0.990332542620729));
#13055=CARTESIAN_POINT('Ctrl Pts',(0.242834539687907,-0.04763,-0.989696097314));
#13056=CARTESIAN_POINT('',(0.528110872004958,-0.04763,-0.871530771444223));
#13057=CARTESIAN_POINT('Origin',(0.,-0.04763,0.));
#13058=CARTESIAN_POINT('',(0.871530771444223,-0.04763,-0.528110872004958));
#13059=CARTESIAN_POINT('Ctrl Pts',(0.528110872004958,-0.0476300000000001,
-0.871530771444223));
#13060=CARTESIAN_POINT('Ctrl Pts',(0.530395067942936,-0.0609922781173484,
-0.870146645090731));
#13061=CARTESIAN_POINT('Ctrl Pts',(0.533674141594226,-0.0742967091364493,
-0.868149331745851));
#13062=CARTESIAN_POINT('Ctrl Pts',(0.54708917182331,-0.115492077056649,
-0.85981294420286));
#13063=CARTESIAN_POINT('Ctrl Pts',(0.560922177770136,-0.141695629206859,
-0.850993704737257));
#13064=CARTESIAN_POINT('Ctrl Pts',(0.590422647829571,-0.181890537957859,
-0.830754510485543));
#13065=CARTESIAN_POINT('Ctrl Pts',(0.609616703125488,-0.201072148666545,
-0.816896541396381));
#13066=CARTESIAN_POINT('Ctrl Pts',(0.641117951819998,-0.223955109275652,
-0.792310597819928));
#13067=CARTESIAN_POINT('Ctrl Pts',(0.657208095763053,-0.232742381310829,
-0.779109323683612));
#13068=CARTESIAN_POINT('Ctrl Pts',(0.68964083160521,-0.244234834628584,
-0.750552691816206));
#13069=CARTESIAN_POINT('Ctrl Pts',(0.705971972091755,-0.246942143572133,
-0.735185187071673));
#13070=CARTESIAN_POINT('Ctrl Pts',(0.735185187071673,-0.246942143572133,
-0.705971972091754));
#13071=CARTESIAN_POINT('Ctrl Pts',(0.750552691816206,-0.244234834628584,
-0.68964083160521));
#13072=CARTESIAN_POINT('Ctrl Pts',(0.779109323683612,-0.232742381310829,
-0.657208095763053));
#13073=CARTESIAN_POINT('Ctrl Pts',(0.792310597819928,-0.223955109275652,
-0.641117951819998));
#13074=CARTESIAN_POINT('Ctrl Pts',(0.816896541396381,-0.201072148666545,
-0.609616703125488));
#13075=CARTESIAN_POINT('Ctrl Pts',(0.830754510485543,-0.181890537957859,
-0.590422647829571));
#13076=CARTESIAN_POINT('Ctrl Pts',(0.850993704737257,-0.141695629206859,
-0.560922177770136));
#13077=CARTESIAN_POINT('Ctrl Pts',(0.85981294420286,-0.115492077056649,
-0.54708917182331));
#13078=CARTESIAN_POINT('Ctrl Pts',(0.868149331745851,-0.0742967091364493,
-0.533674141594226));
#13079=CARTESIAN_POINT('Ctrl Pts',(0.870146645090731,-0.0609922781173484,
-0.530395067942936));
#13080=CARTESIAN_POINT('Ctrl Pts',(0.871530771444223,-0.0476300000000001,
-0.528110872004958));
#13081=CARTESIAN_POINT('',(0.989696097314,-0.04763,-0.242834539687906));
#13082=CARTESIAN_POINT('Origin',(0.,-0.04763,0.));
#13083=CARTESIAN_POINT('',(0.989696097314,-0.04763,0.242834539687906));
#13084=CARTESIAN_POINT('Ctrl Pts',(0.989696097314,-0.04763,-0.242834539687907));
#13085=CARTESIAN_POINT('Ctrl Pts',(0.990332542620729,-0.0609922781173483,
-0.24024064412003));
#13086=CARTESIAN_POINT('Ctrl Pts',(0.991238884025248,-0.0742967091364493,
-0.236509675094874));
#13087=CARTESIAN_POINT('Ctrl Pts',(0.994830026707808,-0.115492077056649,
-0.221129100087819));
#13088=CARTESIAN_POINT('Ctrl Pts',(0.998375294985966,-0.141695629206859,
-0.205111543747588));
#13089=CARTESIAN_POINT('Ctrl Pts',(1.00492400591205,-0.181890537957859,
-0.169940289819232));
#13090=CARTESIAN_POINT('Ctrl Pts',(1.00869718865384,-0.201072148666545,
-0.1465689792446));
#13091=CARTESIAN_POINT('Ctrl Pts',(1.01358704779679,-0.223955109275652,
-0.106909345252087));
#13092=CARTESIAN_POINT('Ctrl Pts',(1.0156297872271,-0.232742381310829,-0.0861971848975942));
#13093=CARTESIAN_POINT('Ctrl Pts',(1.01837060663223,-0.244234834628584,
-0.0430711894098823));
#13094=CARTESIAN_POINT('Ctrl Pts',(1.019052,-0.246942143572133,-0.0206568624125607));
#13095=CARTESIAN_POINT('Ctrl Pts',(1.019052,-0.246942143572133,0.0206568624125607));
#13096=CARTESIAN_POINT('Ctrl Pts',(1.01837060663223,-0.244234834628584,
0.0430711894098823));
#13097=CARTESIAN_POINT('Ctrl Pts',(1.0156297872271,-0.232742381310829,0.0861971848975942));
#13098=CARTESIAN_POINT('Ctrl Pts',(1.01358704779679,-0.223955109275652,
0.106909345252087));
#13099=CARTESIAN_POINT('Ctrl Pts',(1.00869718865384,-0.201072148666545,
0.1465689792446));
#13100=CARTESIAN_POINT('Ctrl Pts',(1.00492400591205,-0.181890537957859,
0.169940289819232));
#13101=CARTESIAN_POINT('Ctrl Pts',(0.998375294985966,-0.141695629206859,
0.205111543747588));
#13102=CARTESIAN_POINT('Ctrl Pts',(0.994830026707808,-0.115492077056649,
0.221129100087819));
#13103=CARTESIAN_POINT('Ctrl Pts',(0.991238884025248,-0.0742967091364492,
0.236509675094874));
#13104=CARTESIAN_POINT('Ctrl Pts',(0.990332542620729,-0.0609922781173483,
0.24024064412003));
#13105=CARTESIAN_POINT('Ctrl Pts',(0.989696097314,-0.04763,0.242834539687907));
#13106=CARTESIAN_POINT('Origin',(0.,-0.04763,0.));
#13107=CARTESIAN_POINT('Origin',(0.,-0.04763,0.));
#13108=CARTESIAN_POINT('',(0.238183666596899,-0.04763,0.951592097314));
#13109=CARTESIAN_POINT('Origin',(0.,-0.04763,0.));
#13110=CARTESIAN_POINT('Origin',(-1.94289029309402E-16,-0.04763,1.));
#13111=CARTESIAN_POINT('Origin',(-1.94289029309402E-16,0.,1.));
#13112=CARTESIAN_POINT('',(-0.2381836665969,-0.04763,0.951592097314));
#13113=CARTESIAN_POINT('Ctrl Pts',(-0.238183666596899,-0.0476299999999999,
0.951592097314));
#13114=CARTESIAN_POINT('Ctrl Pts',(-0.233157223576062,-0.0740444353928835,
0.952850216871763));
#13115=CARTESIAN_POINT('Ctrl Pts',(-0.223801617934946,-0.0999305678883309,
0.955173119738174));
#13116=CARTESIAN_POINT('Ctrl Pts',(-0.199966927975188,-0.142345102874864,
0.960411259488514));
#13117=CARTESIAN_POINT('Ctrl Pts',(-0.1868781821531,-0.159766064500479,
0.963103647174702));
#13118=CARTESIAN_POINT('Ctrl Pts',(-0.15681442133453,-0.190326085855194,
0.968453058988463));
#13119=CARTESIAN_POINT('Ctrl Pts',(-0.139836317888043,-0.203463743702801,
0.971100730005489));
#13120=CARTESIAN_POINT('Ctrl Pts',(-0.104422493053067,-0.224161999508995,
0.975530745318961));
#13121=CARTESIAN_POINT('Ctrl Pts',(-0.0842175114474176,-0.232861760990032,
0.977553872336861));
#13122=CARTESIAN_POINT('Ctrl Pts',(-0.0421062857595701,-0.244251601209411,
0.980270995488453));
#13123=CARTESIAN_POINT('Ctrl Pts',(-0.0201990724523197,-0.246942143572133,
0.980948));
#13124=CARTESIAN_POINT('Ctrl Pts',(0.020199072452319,-0.246942143572133,
0.980948));
#13125=CARTESIAN_POINT('Ctrl Pts',(0.0421062857595694,-0.244251601209411,
0.980270995488454));
#13126=CARTESIAN_POINT('Ctrl Pts',(0.0842175114474169,-0.232861760990032,
0.977553872336861));
#13127=CARTESIAN_POINT('Ctrl Pts',(0.104422493053067,-0.224161999508995,
0.975530745318961));
#13128=CARTESIAN_POINT('Ctrl Pts',(0.139836317888042,-0.203463743702801,
0.971100730005489));
#13129=CARTESIAN_POINT('Ctrl Pts',(0.15681442133453,-0.190326085855194,
0.968453058988463));
#13130=CARTESIAN_POINT('Ctrl Pts',(0.1868781821531,-0.15976606450048,0.963103647174702));
#13131=CARTESIAN_POINT('Ctrl Pts',(0.199966927975188,-0.142345102874864,
0.960411259488514));
#13132=CARTESIAN_POINT('Ctrl Pts',(0.223801617934945,-0.0999305678883309,
0.955173119738174));
#13133=CARTESIAN_POINT('Ctrl Pts',(0.233157223576061,-0.0740444353928835,
0.952850216871763));
#13134=CARTESIAN_POINT('Ctrl Pts',(0.238183666596899,-0.0476299999999999,
0.951592097314));
#13135=CARTESIAN_POINT('Origin',(-1.94289029309402E-16,-0.04763,1.));
#13136=CARTESIAN_POINT('Origin',(0.,-0.04763,0.));
#13137=CARTESIAN_POINT('',(-0.504455939115715,-0.04763,0.841298510752802));
#13138=CARTESIAN_POINT('Origin',(0.,-0.04763,0.));
#13139=CARTESIAN_POINT('Origin',(-0.707106781186548,-0.04763,0.707106781186547));
#13140=CARTESIAN_POINT('Origin',(-0.707106781186548,0.,0.707106781186547));
#13141=CARTESIAN_POINT('',(-0.841298510752802,-0.04763,0.504455939115715));
#13142=CARTESIAN_POINT('Ctrl Pts',(-0.841298510752802,-0.04763,0.504455939115715));
#13143=CARTESIAN_POINT('Ctrl Pts',(-0.838633903678357,-0.0740444353928835,
0.508899795931835));
#13144=CARTESIAN_POINT('Ctrl Pts',(-0.833661031856294,-0.0999305678883309,
0.517157748491652));
#13145=CARTESIAN_POINT('Ctrl Pts',(-0.820511285096538,-0.142345102874864,
0.537715343527944));
#13146=CARTESIAN_POINT('Ctrl Pts',(-0.813159949759,-0.159766064500479,0.548874290046456));
#13147=CARTESIAN_POINT('Ctrl Pts',(-0.795684265985089,-0.190326085855194,
0.573915184558107));
#13148=CARTESIAN_POINT('Ctrl Pts',(-0.78555112003688,-0.203463743702801,
0.587792702767295));
#13149=CARTESIAN_POINT('Ctrl Pts',(-0.763642258217233,-0.224161999508995,
0.615966552324775));
#13150=CARTESIAN_POINT('Ctrl Pts',(-0.750785745543687,-0.232861760990032,
0.631684198665438));
#13151=CARTESIAN_POINT('Ctrl Pts',(-0.722929908501543,-0.244251601209411,
0.663382628119203));
#13152=CARTESIAN_POINT('Ctrl Pts',(-0.707917883896095,-0.246942143572133,
0.679352081686668));
#13153=CARTESIAN_POINT('Ctrl Pts',(-0.679352081686668,-0.246942143572133,
0.707917883896095));
#13154=CARTESIAN_POINT('Ctrl Pts',(-0.663382628119203,-0.244251601209411,
0.722929908501544));
#13155=CARTESIAN_POINT('Ctrl Pts',(-0.631684198665438,-0.232861760990031,
0.750785745543687));
#13156=CARTESIAN_POINT('Ctrl Pts',(-0.615966552324775,-0.224161999508995,
0.763642258217233));
#13157=CARTESIAN_POINT('Ctrl Pts',(-0.587792702767295,-0.203463743702801,
0.78555112003688));
#13158=CARTESIAN_POINT('Ctrl Pts',(-0.573915184558107,-0.190326085855194,
0.795684265985088));
#13159=CARTESIAN_POINT('Ctrl Pts',(-0.548874290046456,-0.159766064500479,
0.813159949759));
#13160=CARTESIAN_POINT('Ctrl Pts',(-0.537715343527944,-0.142345102874864,
0.820511285096538));
#13161=CARTESIAN_POINT('Ctrl Pts',(-0.517157748491652,-0.0999305678883309,
0.833661031856294));
#13162=CARTESIAN_POINT('Ctrl Pts',(-0.508899795931835,-0.0740444353928835,
0.838633903678357));
#13163=CARTESIAN_POINT('Ctrl Pts',(-0.504455939115716,-0.04763,0.841298510752801));
#13164=CARTESIAN_POINT('Origin',(-0.707106781186548,-0.04763,0.707106781186547));
#13165=CARTESIAN_POINT('Origin',(0.,-0.04763,0.));
#13166=CARTESIAN_POINT('',(-0.951592097314,-0.04763,0.238183666596899));
#13167=CARTESIAN_POINT('Origin',(0.,-0.04763,0.));
#13168=CARTESIAN_POINT('Origin',(-1.,-0.04763,-1.11022302462516E-16));
#13169=CARTESIAN_POINT('Origin',(-1.,0.,-1.11022302462516E-16));
#13170=CARTESIAN_POINT('',(-0.951592097314,-0.04763,-0.2381836665969));
#13171=CARTESIAN_POINT('',(-0.980948,-0.246942143572133,1.08514323328844E-18));
#13172=CARTESIAN_POINT('Ctrl Pts',(-0.951592097314,-0.04763,-0.238183666596899));
#13173=CARTESIAN_POINT('Ctrl Pts',(-0.952850216871763,-0.0740444353928835,
-0.233157223576062));
#13174=CARTESIAN_POINT('Ctrl Pts',(-0.955173119738174,-0.0999305678883309,
-0.223801617934946));
#13175=CARTESIAN_POINT('Ctrl Pts',(-0.960411259488514,-0.142345102874864,
-0.199966927975188));
#13176=CARTESIAN_POINT('Ctrl Pts',(-0.963103647174702,-0.159766064500479,
-0.1868781821531));
#13177=CARTESIAN_POINT('Ctrl Pts',(-0.968453058988463,-0.190326085855194,
-0.15681442133453));
#13178=CARTESIAN_POINT('Ctrl Pts',(-0.971100730005489,-0.203463743702801,
-0.139836317888043));
#13179=CARTESIAN_POINT('Ctrl Pts',(-0.975530745318961,-0.224161999508995,
-0.104422493053067));
#13180=CARTESIAN_POINT('Ctrl Pts',(-0.977553872336861,-0.232861760990032,
-0.0842175114474175));
#13181=CARTESIAN_POINT('Ctrl Pts',(-0.980270995488453,-0.244251601209411,
-0.0421062857595699));
#13182=CARTESIAN_POINT('Ctrl Pts',(-0.980948,-0.246942143572133,-0.0201990724523195));
#13183=CARTESIAN_POINT('Ctrl Pts',(-0.980948,-0.246942143572133,-1.17961196366423E-16));
#13184=CARTESIAN_POINT('Origin',(-1.,-0.04763,-1.11022302462516E-16));
#13185=CARTESIAN_POINT('Ctrl Pts',(-0.980948,-0.246942143572133,-1.17961196366423E-16));
#13186=CARTESIAN_POINT('Ctrl Pts',(-0.980948,-0.246942143572133,0.0201990724523192));
#13187=CARTESIAN_POINT('Ctrl Pts',(-0.980270995488453,-0.244251601209411,
0.0421062857595695));
#13188=CARTESIAN_POINT('Ctrl Pts',(-0.977553872336861,-0.232861760990032,
0.0842175114474169));
#13189=CARTESIAN_POINT('Ctrl Pts',(-0.975530745318961,-0.224161999508995,
0.104422493053066));
#13190=CARTESIAN_POINT('Ctrl Pts',(-0.971100730005489,-0.203463743702801,
0.139836317888042));
#13191=CARTESIAN_POINT('Ctrl Pts',(-0.968453058988463,-0.190326085855194,
0.15681442133453));
#13192=CARTESIAN_POINT('Ctrl Pts',(-0.963103647174702,-0.15976606450048,
0.1868781821531));
#13193=CARTESIAN_POINT('Ctrl Pts',(-0.960411259488514,-0.142345102874864,
0.199966927975188));
#13194=CARTESIAN_POINT('Ctrl Pts',(-0.955173119738174,-0.099930567888331,
0.223801617934945));
#13195=CARTESIAN_POINT('Ctrl Pts',(-0.952850216871763,-0.0740444353928835,
0.233157223576061));
#13196=CARTESIAN_POINT('Ctrl Pts',(-0.951592097314,-0.04763,0.238183666596899));
#13197=CARTESIAN_POINT('Origin',(0.,-0.04763,0.));
#13198=CARTESIAN_POINT('',(-0.841298510752802,-0.04763,-0.504455939115715));
#13199=CARTESIAN_POINT('Origin',(0.,-0.04763,0.));
#13200=CARTESIAN_POINT('Origin',(-0.707106781186547,-0.04763,-0.707106781186548));
#13201=CARTESIAN_POINT('Origin',(-0.707106781186547,0.,-0.707106781186548));
#13202=CARTESIAN_POINT('',(-0.504455939115715,-0.04763,-0.841298510752802));
#13203=CARTESIAN_POINT('Ctrl Pts',(-0.504455939115715,-0.04763,-0.841298510752802));
#13204=CARTESIAN_POINT('Ctrl Pts',(-0.508899795931835,-0.0740444353928835,
-0.838633903678357));
#13205=CARTESIAN_POINT('Ctrl Pts',(-0.517157748491652,-0.0999305678883309,
-0.833661031856294));
#13206=CARTESIAN_POINT('Ctrl Pts',(-0.537715343527944,-0.142345102874864,
-0.820511285096538));
#13207=CARTESIAN_POINT('Ctrl Pts',(-0.548874290046456,-0.159766064500479,
-0.813159949759));
#13208=CARTESIAN_POINT('Ctrl Pts',(-0.573915184558107,-0.190326085855194,
-0.795684265985089));
#13209=CARTESIAN_POINT('Ctrl Pts',(-0.587792702767295,-0.203463743702801,
-0.78555112003688));
#13210=CARTESIAN_POINT('Ctrl Pts',(-0.615966552324775,-0.224161999508995,
-0.763642258217233));
#13211=CARTESIAN_POINT('Ctrl Pts',(-0.631684198665438,-0.232861760990032,
-0.750785745543687));
#13212=CARTESIAN_POINT('Ctrl Pts',(-0.663382628119203,-0.244251601209411,
-0.722929908501543));
#13213=CARTESIAN_POINT('Ctrl Pts',(-0.679352081686668,-0.246942143572133,
-0.707917883896095));
#13214=CARTESIAN_POINT('Ctrl Pts',(-0.707917883896095,-0.246942143572133,
-0.679352081686668));
#13215=CARTESIAN_POINT('Ctrl Pts',(-0.722929908501543,-0.244251601209411,
-0.663382628119203));
#13216=CARTESIAN_POINT('Ctrl Pts',(-0.750785745543687,-0.232861760990032,
-0.631684198665439));
#13217=CARTESIAN_POINT('Ctrl Pts',(-0.763642258217232,-0.224161999508995,
-0.615966552324775));
#13218=CARTESIAN_POINT('Ctrl Pts',(-0.78555112003688,-0.203463743702801,
-0.587792702767295));
#13219=CARTESIAN_POINT('Ctrl Pts',(-0.795684265985088,-0.190326085855194,
-0.573915184558107));
#13220=CARTESIAN_POINT('Ctrl Pts',(-0.813159949759,-0.15976606450048,-0.548874290046456));
#13221=CARTESIAN_POINT('Ctrl Pts',(-0.820511285096538,-0.142345102874864,
-0.537715343527944));
#13222=CARTESIAN_POINT('Ctrl Pts',(-0.833661031856294,-0.0999305678883311,
-0.517157748491652));
#13223=CARTESIAN_POINT('Ctrl Pts',(-0.838633903678357,-0.0740444353928836,
-0.508899795931835));
#13224=CARTESIAN_POINT('Ctrl Pts',(-0.841298510752801,-0.04763,-0.504455939115715));
#13225=CARTESIAN_POINT('Origin',(-0.707106781186547,-0.04763,-0.707106781186548));
#13226=CARTESIAN_POINT('Origin',(0.,-0.04763,0.));
#13227=CARTESIAN_POINT('',(-0.238183666596899,-0.04763,-0.951592097314));
#13228=CARTESIAN_POINT('Origin',(0.,-0.04763,0.));
#13229=CARTESIAN_POINT('Origin',(5.55111512312578E-17,-0.04763,-1.));
#13230=CARTESIAN_POINT('Origin',(5.55111512312578E-17,0.,-1.));
#13231=CARTESIAN_POINT('',(0.238183666596899,-0.04763,-0.951592097314));
#13232=CARTESIAN_POINT('Ctrl Pts',(0.238183666596899,-0.04763,-0.951592097314));
#13233=CARTESIAN_POINT('Ctrl Pts',(0.233157223576062,-0.0740444353928835,
-0.952850216871763));
#13234=CARTESIAN_POINT('Ctrl Pts',(0.223801617934946,-0.099930567888331,
-0.955173119738174));
#13235=CARTESIAN_POINT('Ctrl Pts',(0.199966927975188,-0.142345102874864,
-0.960411259488514));
#13236=CARTESIAN_POINT('Ctrl Pts',(0.1868781821531,-0.15976606450048,-0.963103647174702));
#13237=CARTESIAN_POINT('Ctrl Pts',(0.15681442133453,-0.190326085855194,
-0.968453058988463));
#13238=CARTESIAN_POINT('Ctrl Pts',(0.139836317888042,-0.203463743702801,
-0.971100730005489));
#13239=CARTESIAN_POINT('Ctrl Pts',(0.104422493053067,-0.224161999508995,
-0.975530745318961));
#13240=CARTESIAN_POINT('Ctrl Pts',(0.0842175114474173,-0.232861760990032,
-0.977553872336861));
#13241=CARTESIAN_POINT('Ctrl Pts',(0.0421062857595698,-0.244251601209411,
-0.980270995488453));
#13242=CARTESIAN_POINT('Ctrl Pts',(0.0201990724523194,-0.246942143572133,
-0.980948));
#13243=CARTESIAN_POINT('Ctrl Pts',(-0.0201990724523193,-0.246942143572133,
-0.980948));
#13244=CARTESIAN_POINT('Ctrl Pts',(-0.0421062857595697,-0.244251601209411,
-0.980270995488453));
#13245=CARTESIAN_POINT('Ctrl Pts',(-0.0842175114474171,-0.232861760990032,
-0.977553872336861));
#13246=CARTESIAN_POINT('Ctrl Pts',(-0.104422493053067,-0.224161999508995,
-0.975530745318961));
#13247=CARTESIAN_POINT('Ctrl Pts',(-0.139836317888042,-0.203463743702801,
-0.971100730005489));
#13248=CARTESIAN_POINT('Ctrl Pts',(-0.15681442133453,-0.190326085855194,
-0.968453058988463));
#13249=CARTESIAN_POINT('Ctrl Pts',(-0.1868781821531,-0.15976606450048,-0.963103647174702));
#13250=CARTESIAN_POINT('Ctrl Pts',(-0.199966927975188,-0.142345102874864,
-0.960411259488514));
#13251=CARTESIAN_POINT('Ctrl Pts',(-0.223801617934945,-0.099930567888331,
-0.955173119738174));
#13252=CARTESIAN_POINT('Ctrl Pts',(-0.233157223576062,-0.0740444353928835,
-0.952850216871763));
#13253=CARTESIAN_POINT('Ctrl Pts',(-0.238183666596899,-0.0476299999999999,
-0.951592097314));
#13254=CARTESIAN_POINT('Origin',(5.55111512312578E-17,-0.04763,-1.));
#13255=CARTESIAN_POINT('Origin',(0.,-0.04763,0.));
#13256=CARTESIAN_POINT('',(0.504455939115715,-0.04763,-0.841298510752802));
#13257=CARTESIAN_POINT('Origin',(0.,-0.04763,0.));
#13258=CARTESIAN_POINT('Origin',(0.707106781186548,-0.04763,-0.707106781186547));
#13259=CARTESIAN_POINT('Origin',(0.707106781186548,0.,-0.707106781186547));
#13260=CARTESIAN_POINT('',(0.841298510752802,-0.04763,-0.504455939115715));
#13261=CARTESIAN_POINT('Ctrl Pts',(0.841298510752802,-0.04763,-0.504455939115715));
#13262=CARTESIAN_POINT('Ctrl Pts',(0.838633903678357,-0.0740444353928835,
-0.508899795931835));
#13263=CARTESIAN_POINT('Ctrl Pts',(0.833661031856294,-0.0999305678883309,
-0.517157748491652));
#13264=CARTESIAN_POINT('Ctrl Pts',(0.820511285096538,-0.142345102874864,
-0.537715343527944));
#13265=CARTESIAN_POINT('Ctrl Pts',(0.813159949759,-0.159766064500479,-0.548874290046456));
#13266=CARTESIAN_POINT('Ctrl Pts',(0.795684265985088,-0.190326085855194,
-0.573915184558107));
#13267=CARTESIAN_POINT('Ctrl Pts',(0.78555112003688,-0.203463743702801,
-0.587792702767295));
#13268=CARTESIAN_POINT('Ctrl Pts',(0.763642258217233,-0.224161999508995,
-0.615966552324775));
#13269=CARTESIAN_POINT('Ctrl Pts',(0.750785745543687,-0.232861760990032,
-0.631684198665438));
#13270=CARTESIAN_POINT('Ctrl Pts',(0.722929908501543,-0.244251601209411,
-0.663382628119203));
#13271=CARTESIAN_POINT('Ctrl Pts',(0.707917883896095,-0.246942143572133,
-0.679352081686668));
#13272=CARTESIAN_POINT('Ctrl Pts',(0.679352081686668,-0.246942143572133,
-0.707917883896095));
#13273=CARTESIAN_POINT('Ctrl Pts',(0.663382628119203,-0.244251601209411,
-0.722929908501543));
#13274=CARTESIAN_POINT('Ctrl Pts',(0.631684198665438,-0.232861760990032,
-0.750785745543687));
#13275=CARTESIAN_POINT('Ctrl Pts',(0.615966552324775,-0.224161999508995,
-0.763642258217232));
#13276=CARTESIAN_POINT('Ctrl Pts',(0.587792702767295,-0.203463743702801,
-0.78555112003688));
#13277=CARTESIAN_POINT('Ctrl Pts',(0.573915184558107,-0.190326085855194,
-0.795684265985088));
#13278=CARTESIAN_POINT('Ctrl Pts',(0.548874290046456,-0.159766064500479,
-0.813159949759));
#13279=CARTESIAN_POINT('Ctrl Pts',(0.537715343527944,-0.142345102874864,
-0.820511285096538));
#13280=CARTESIAN_POINT('Ctrl Pts',(0.517157748491652,-0.099930567888331,
-0.833661031856294));
#13281=CARTESIAN_POINT('Ctrl Pts',(0.508899795931835,-0.0740444353928835,
-0.838633903678357));
#13282=CARTESIAN_POINT('Ctrl Pts',(0.504455939115715,-0.04763,-0.841298510752801));
#13283=CARTESIAN_POINT('Origin',(0.707106781186548,-0.04763,-0.707106781186547));
#13284=CARTESIAN_POINT('Origin',(0.,-0.166705,0.));
#13285=CARTESIAN_POINT('',(-0.980948,-0.28578,1.20131482833E-16));
#13286=CARTESIAN_POINT('Origin',(0.,-0.28578,0.));
#13287=CARTESIAN_POINT('',(-0.980948,-0.166705,1.20131482833E-16));
#13288=CARTESIAN_POINT('',(0.951592097314,-0.04763,0.238183666596899));
#13289=CARTESIAN_POINT('Origin',(0.,-0.04763,0.));
#13290=CARTESIAN_POINT('',(0.951592097314,-0.04763,-0.238183666596899));
#13291=CARTESIAN_POINT('Ctrl Pts',(0.951592097314,-0.04763,0.238183666596899));
#13292=CARTESIAN_POINT('Ctrl Pts',(0.952850216871763,-0.0740444353928835,
0.233157223576062));
#13293=CARTESIAN_POINT('Ctrl Pts',(0.955173119738174,-0.099930567888331,
0.223801617934945));
#13294=CARTESIAN_POINT('Ctrl Pts',(0.960411259488514,-0.142345102874864,
0.199966927975188));
#13295=CARTESIAN_POINT('Ctrl Pts',(0.963103647174702,-0.15976606450048,
0.1868781821531));
#13296=CARTESIAN_POINT('Ctrl Pts',(0.968453058988463,-0.190326085855194,
0.15681442133453));
#13297=CARTESIAN_POINT('Ctrl Pts',(0.971100730005489,-0.203463743702801,
0.139836317888042));
#13298=CARTESIAN_POINT('Ctrl Pts',(0.975530745318961,-0.224161999508995,
0.104422493053067));
#13299=CARTESIAN_POINT('Ctrl Pts',(0.977553872336861,-0.232861760990032,
0.0842175114474172));
#13300=CARTESIAN_POINT('Ctrl Pts',(0.980270995488453,-0.244251601209411,
0.0421062857595697));
#13301=CARTESIAN_POINT('Ctrl Pts',(0.980948,-0.246942143572133,0.0201990724523194));
#13302=CARTESIAN_POINT('Ctrl Pts',(0.980948,-0.246942143572133,-0.0201990724523194));
#13303=CARTESIAN_POINT('Ctrl Pts',(0.980270995488453,-0.244251601209411,
-0.0421062857595697));
#13304=CARTESIAN_POINT('Ctrl Pts',(0.977553872336861,-0.232861760990032,
-0.0842175114474172));
#13305=CARTESIAN_POINT('Ctrl Pts',(0.975530745318961,-0.224161999508995,
-0.104422493053067));
#13306=CARTESIAN_POINT('Ctrl Pts',(0.971100730005489,-0.203463743702801,
-0.139836317888042));
#13307=CARTESIAN_POINT('Ctrl Pts',(0.968453058988463,-0.190326085855194,
-0.15681442133453));
#13308=CARTESIAN_POINT('Ctrl Pts',(0.963103647174702,-0.15976606450048,
-0.1868781821531));
#13309=CARTESIAN_POINT('Ctrl Pts',(0.960411259488514,-0.142345102874864,
-0.199966927975188));
#13310=CARTESIAN_POINT('Ctrl Pts',(0.955173119738174,-0.099930567888331,
-0.223801617934945));
#13311=CARTESIAN_POINT('Ctrl Pts',(0.952850216871763,-0.0740444353928835,
-0.233157223576062));
#13312=CARTESIAN_POINT('Ctrl Pts',(0.951592097314,-0.0476299999999999,-0.238183666596899));
#13313=CARTESIAN_POINT('Origin',(0.,-0.04763,0.));
#13314=CARTESIAN_POINT('Origin',(0.,-0.04763,0.));
#13315=CARTESIAN_POINT('Origin',(1.,-0.04763,0.));
#13316=CARTESIAN_POINT('Origin',(1.,0.,0.));
#13317=CARTESIAN_POINT('Origin',(1.,-0.04763,0.));
#13318=CARTESIAN_POINT('Origin',(0.,-0.28578,0.));
#13319=CARTESIAN_POINT('Origin',(0.,-0.04763,0.));
#13774=UNCERTAINTY_MEASURE_WITH_UNIT(LENGTH_MEASURE(0.001),#13822,
'DISTANCE_ACCURACY_VALUE',
'Maximum model space distance between geometric entities at asserted c
onnectivities');
#13782=UNCERTAINTY_MEASURE_WITH_UNIT(LENGTH_MEASURE(0.001),#13822,
'DISTANCE_ACCURACY_VALUE',
'Maximum model space distance between geometric entities at asserted c
onnectivities');
#13813=(
GEOMETRIC_REPRESENTATION_CONTEXT(3)
GLOBAL_UNCERTAINTY_ASSIGNED_CONTEXT((#13774))
GLOBAL_UNIT_ASSIGNED_CONTEXT((#13822,#13824,#13825))
REPRESENTATION_CONTEXT('','3D')
);
#13821=(
GEOMETRIC_REPRESENTATION_CONTEXT(3)
GLOBAL_UNCERTAINTY_ASSIGNED_CONTEXT((#13782))
GLOBAL_UNIT_ASSIGNED_CONTEXT((#13822,#13824,#13825))
REPRESENTATION_CONTEXT('','3D')
);
#13822=(
LENGTH_UNIT()
NAMED_UNIT(*)
SI_UNIT(.CENTI.,.METRE.)
);
#13824=(
NAMED_UNIT(*)
PLANE_ANGLE_UNIT()
SI_UNIT($,.RADIAN.)
);
#13825=(
NAMED_UNIT(*)
SI_UNIT($,.STERADIAN.)
SOLID_ANGLE_UNIT()
);
#13856=SHAPE_DEFINITION_REPRESENTATION(#13894,#14026);
#13894=PRODUCT_DEFINITION_SHAPE('',$,#14065);
#14026=SHAPE_REPRESENTATION('',(#8541),#13813);
#14034=PRODUCT_DEFINITION_CONTEXT('part definition',#14150,'design');
#14065=PRODUCT_DEFINITION('Cage','Cage',#14103,#14034);
#14103=PRODUCT_DEFINITION_FORMATION('',$,#14182);
#14150=APPLICATION_CONTEXT(
'Core Data for Automotive Mechanical Design Process');
#14151=PRODUCT_CONTEXT('part definition',#14150,'mechanical');
#14182=PRODUCT('Cage','Cage','Cage',(#14151));
#14190=PRESENTATION_STYLE_ASSIGNMENT((#14195));
#14195=SURFACE_STYLE_USAGE(.BOTH.,#14200);
#14200=SURFACE_SIDE_STYLE('',(#14205));
#14205=SURFACE_STYLE_FILL_AREA(#14210);
#14210=FILL_AREA_STYLE('Steel - Satin',(#14215));
#14215=FILL_AREA_STYLE_COLOUR('Steel - Satin',#14220);
#14220=COLOUR_RGB('Steel - Satin',0.627450980392157,0.627450980392157,0.627450980392157);
ENDSEC;
END-ISO-10303-21;
